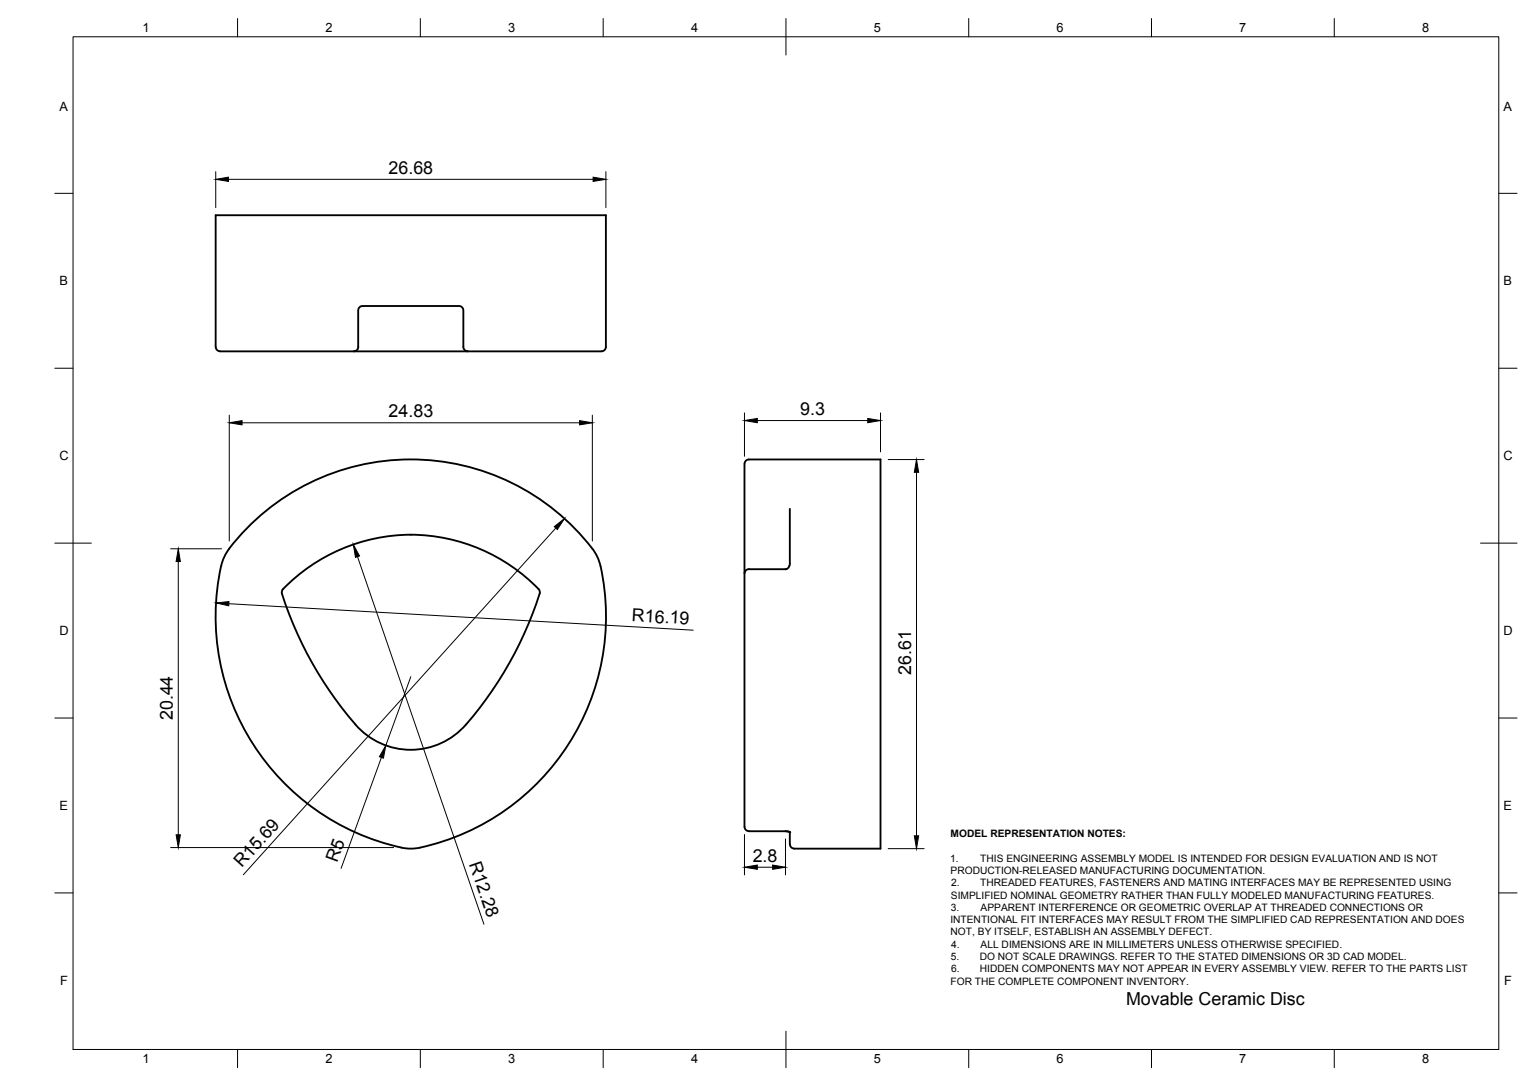
ISO-10303-21;
HEADER;
/* Generated by software containing ST-Developer
 * from STEP Tools, Inc. (www.steptools.com) 
 */

FILE_DESCRIPTION(
/* description */ ('STEP AP214'),
/* implementation_level */ '2;1');

FILE_NAME(
/* name */ 'Movable Ceramic Disc.step',
/* time_stamp */ '2026-10-06T00:19:40-07:00',
/* author */ (''),
/* organization */ (''),
/* preprocessor_version */ 'ST-DEVELOPER v20.2',
/* originating_system */ 'Autodesk Translation Framework v15.15.0.0',
/* authorisation */ '');

FILE_SCHEMA (('AUTOMOTIVE_DESIGN { 1 0 10303 214 3 1 1 }'));
ENDSEC;

DATA;
#10=MECHANICAL_DESIGN_GEOMETRIC_PRESENTATION_REPRESENTATION('',(#2071),#98302);
#411=TOROIDAL_SURFACE('',#38089,13.016744254,0.3);
#412=TOROIDAL_SURFACE('',#38103,25.2066723663,0.5);
#413=TOROIDAL_SURFACE('',#38106,11.7773059952,0.5);
#414=TOROIDAL_SURFACE('',#38114,4.5,0.5);
#415=TOROIDAL_SURFACE('',#38119,25.2066723663,0.5);
#416=TOROIDAL_SURFACE('',#38123,4.5,0.5);
#417=TOROIDAL_SURFACE('',#38131,11.7773059952,0.5);
#418=TOROIDAL_SURFACE('',#38142,13.616744254,0.3);
#419=TOROIDAL_SURFACE('',#38173,13.616744254,0.3);
#420=TOROIDAL_SURFACE('',#38197,13.7462109523,0.3);
#421=TOROIDAL_SURFACE('',#38202,2.8,0.3);
#422=TOROIDAL_SURFACE('',#38207,13.7462109523,0.3);
#423=TOROIDAL_SURFACE('',#38229,0.6,0.3);
#424=TOROIDAL_SURFACE('',#38232,13.016744254,0.3);
#425=TOROIDAL_SURFACE('',#38235,0.6,0.3);
#426=TOROIDAL_SURFACE('',#38243,0.6,0.3);
#427=TOROIDAL_SURFACE('',#38245,0.6,0.3);
#428=TOROIDAL_SURFACE('',#38253,0.6,0.3);
#429=TOROIDAL_SURFACE('',#38256,13.1462109523,0.3);
#430=TOROIDAL_SURFACE('',#38259,2.2,0.3);
#431=TOROIDAL_SURFACE('',#38262,13.1462109523,0.3);
#432=TOROIDAL_SURFACE('',#38265,0.6,0.3);
#433=TOROIDAL_SURFACE('',#38283,15.8875296363,0.3);
#434=TOROIDAL_SURFACE('',#38290,15.8875296363,0.3);
#435=TOROIDAL_SURFACE('',#38294,2.7,0.3);
#436=TOROIDAL_SURFACE('',#38307,15.8875296363,0.3);
#437=TOROIDAL_SURFACE('',#38312,15.8875296363,0.3);
#438=TOROIDAL_SURFACE('',#38317,2.7,0.3);
#439=TOROIDAL_SURFACE('',#38322,2.7,0.3);
#440=TOROIDAL_SURFACE('',#38336,15.3875296363,0.3);
#441=TOROIDAL_SURFACE('',#38338,15.3875296363,0.3);
#442=TOROIDAL_SURFACE('',#38342,15.3875296363,0.3);
#706=ELLIPSE('',#38289,0.298848923957396,0.296905362261884);
#707=ELLIPSE('',#38314,0.2988489185537,0.296905422816142);
#708=ELLIPSE('',#38324,0.298848919017662,0.29690542389071);
#709=ELLIPSE('',#38343,0.298849404757611,0.296905780207238);
#847=SPHERICAL_SURFACE('',#38146,0.3);
#848=SPHERICAL_SURFACE('',#38154,0.3);
#849=SPHERICAL_SURFACE('',#38166,0.3);
#850=SPHERICAL_SURFACE('',#38177,0.3);
#851=SPHERICAL_SURFACE('',#38195,0.3);
#852=SPHERICAL_SURFACE('',#38214,0.3);
#853=SPHERICAL_SURFACE('',#38274,0.3);
#854=SPHERICAL_SURFACE('',#38278,0.3);
#855=SPHERICAL_SURFACE('',#38298,0.3);
#856=SPHERICAL_SURFACE('',#38303,0.3);
#857=SPHERICAL_SURFACE('',#38327,0.3);
#858=SPHERICAL_SURFACE('',#38331,0.3);
#1242=B_SPLINE_SURFACE_WITH_KNOTS('',4,5,((#95885,#95886,#95887,#95888,
#95889,#95890),(#95891,#95892,#95893,#95894,#95895,#95896),(#95897,#95898,
#95899,#95900,#95901,#95902),(#95903,#95904,#95905,#95906,#95907,#95908),
(#95909,#95910,#95911,#95912,#95913,#95914)),.UNSPECIFIED.,.F.,.F.,.F.,
(5,5),(6,6),(0.,1.12670233583),(0.,0.3),.UNSPECIFIED.);
#1243=B_SPLINE_SURFACE_WITH_KNOTS('',4,5,((#96049,#96050,#96051,#96052,
#96053,#96054),(#96055,#96056,#96057,#96058,#96059,#96060),(#96061,#96062,
#96063,#96064,#96065,#96066),(#96067,#96068,#96069,#96070,#96071,#96072),
(#96073,#96074,#96075,#96076,#96077,#96078)),.UNSPECIFIED.,.F.,.F.,.F.,
(5,5),(6,6),(0.,1.12670210859),(0.,0.3),.UNSPECIFIED.);
#1244=B_SPLINE_SURFACE_WITH_KNOTS('',5,5,((#96516,#96517,#96518,#96519,
#96520,#96521,#96522,#96523,#96524),(#96525,#96526,#96527,#96528,#96529,
#96530,#96531,#96532,#96533),(#96534,#96535,#96536,#96537,#96538,#96539,
#96540,#96541,#96542),(#96543,#96544,#96545,#96546,#96547,#96548,#96549,
#96550,#96551),(#96552,#96553,#96554,#96555,#96556,#96557,#96558,#96559,
#96560),(#96561,#96562,#96563,#96564,#96565,#96566,#96567,#96568,#96569),
(#96570,#96571,#96572,#96573,#96574,#96575,#96576,#96577,#96578),(#96579,
#96580,#96581,#96582,#96583,#96584,#96585,#96586,#96587),(#96588,#96589,
#96590,#96591,#96592,#96593,#96594,#96595,#96596)),.UNSPECIFIED.,.F.,.F.,
 .F.,(6,3,6),(6,3,6),(1.82800160081,2.29147741959,2.71936718506),(0.,0.15,
0.3),.UNSPECIFIED.);
#1245=B_SPLINE_SURFACE_WITH_KNOTS('',5,5,((#96621,#96622,#96623,#96624,
#96625,#96626),(#96627,#96628,#96629,#96630,#96631,#96632),(#96633,#96634,
#96635,#96636,#96637,#96638),(#96639,#96640,#96641,#96642,#96643,#96644),
(#96645,#96646,#96647,#96648,#96649,#96650),(#96651,#96652,#96653,#96654,
#96655,#96656),(#96657,#96658,#96659,#96660,#96661,#96662),(#96663,#96664,
#96665,#96666,#96667,#96668),(#96669,#96670,#96671,#96672,#96673,#96674)),
 .UNSPECIFIED.,.F.,.F.,.F.,(6,3,6),(6,6),(1.72679799842804,2.34453942473,
2.86671715236056),(0.,0.300030052101964),.UNSPECIFIED.);
#1246=B_SPLINE_SURFACE_WITH_KNOTS('',5,5,((#96715,#96716,#96717,#96718,
#96719,#96720,#96721,#96722,#96723),(#96724,#96725,#96726,#96727,#96728,
#96729,#96730,#96731,#96732),(#96733,#96734,#96735,#96736,#96737,#96738,
#96739,#96740,#96741),(#96742,#96743,#96744,#96745,#96746,#96747,#96748,
#96749,#96750),(#96751,#96752,#96753,#96754,#96755,#96756,#96757,#96758,
#96759),(#96760,#96761,#96762,#96763,#96764,#96765,#96766,#96767,#96768),
(#96769,#96770,#96771,#96772,#96773,#96774,#96775,#96776,#96777),(#96778,
#96779,#96780,#96781,#96782,#96783,#96784,#96785,#96786),(#96787,#96788,
#96789,#96790,#96791,#96792,#96793,#96794,#96795)),.UNSPECIFIED.,.F.,.F.,
 .F.,(6,3,6),(6,3,6),(2.03426195559,2.39548583384,2.92554757),(0.,0.15,
0.3),.UNSPECIFIED.);
#1247=B_SPLINE_SURFACE_WITH_KNOTS('',5,5,((#96840,#96841,#96842,#96843,
#96844,#96845),(#96846,#96847,#96848,#96849,#96850,#96851),(#96852,#96853,
#96854,#96855,#96856,#96857),(#96858,#96859,#96860,#96861,#96862,#96863),
(#96864,#96865,#96866,#96867,#96868,#96869),(#96870,#96871,#96872,#96873,
#96874,#96875),(#96876,#96877,#96878,#96879,#96880,#96881),(#96882,#96883,
#96884,#96885,#96886,#96887),(#96888,#96889,#96890,#96891,#96892,#96893)),
 .UNSPECIFIED.,.F.,.F.,.F.,(6,3,6),(6,6),(1.66562909398,2.17637755312,2.80548129619),
(0.,0.3),.UNSPECIFIED.);
#1248=B_SPLINE_SURFACE_WITH_KNOTS('',5,5,((#96951,#96952,#96953,#96954,
#96955,#96956),(#96957,#96958,#96959,#96960,#96961,#96962),(#96963,#96964,
#96965,#96966,#96967,#96968),(#96969,#96970,#96971,#96972,#96973,#96974),
(#96975,#96976,#96977,#96978,#96979,#96980),(#96981,#96982,#96983,#96984,
#96985,#96986)),.UNSPECIFIED.,.F.,.F.,.F.,(6,6),(6,6),(1.15863824043,1.47670435084),
(0.,0.3),.UNSPECIFIED.);
#1249=B_SPLINE_SURFACE_WITH_KNOTS('',5,5,((#97008,#97009,#97010,#97011,
#97012,#97013),(#97014,#97015,#97016,#97017,#97018,#97019),(#97020,#97021,
#97022,#97023,#97024,#97025),(#97026,#97027,#97028,#97029,#97030,#97031),
(#97032,#97033,#97034,#97035,#97036,#97037),(#97038,#97039,#97040,#97041,
#97042,#97043)),.UNSPECIFIED.,.F.,.F.,.F.,(6,6),(6,6),(1.69754904882,2.01561058189),
(0.,0.3),.UNSPECIFIED.);
#1250=B_SPLINE_SURFACE_WITH_KNOTS('',5,5,((#97079,#97080,#97081,#97082,
#97083,#97084),(#97085,#97086,#97087,#97088,#97089,#97090),(#97091,#97092,
#97093,#97094,#97095,#97096),(#97097,#97098,#97099,#97100,#97101,#97102),
(#97103,#97104,#97105,#97106,#97107,#97108),(#97109,#97110,#97111,#97112,
#97113,#97114),(#97115,#97116,#97117,#97118,#97119,#97120),(#97121,#97122,
#97123,#97124,#97125,#97126),(#97127,#97128,#97129,#97130,#97131,#97132)),
 .UNSPECIFIED.,.F.,.F.,.F.,(6,3,6),(6,6),(1.64809551428,2.25520583962,2.74124708106),
(0.,0.3),.UNSPECIFIED.);
#1251=B_SPLINE_SURFACE_WITH_KNOTS('',5,5,((#97186,#97187,#97188,#97189,
#97190,#97191),(#97192,#97193,#97194,#97195,#97196,#97197),(#97198,#97199,
#97200,#97201,#97202,#97203),(#97204,#97205,#97206,#97207,#97208,#97209),
(#97210,#97211,#97212,#97213,#97214,#97215),(#97216,#97217,#97218,#97219,
#97220,#97221),(#97222,#97223,#97224,#97225,#97226,#97227),(#97228,#97229,
#97230,#97231,#97232,#97233),(#97234,#97235,#97236,#97237,#97238,#97239)),
 .UNSPECIFIED.,.F.,.F.,.F.,(6,3,6),(6,6),(1.62043318117,2.09769319653,2.71358394784),
(0.,0.3),.UNSPECIFIED.);
#1315=FACE_BOUND('',#7442,.T.);
#2003=B_SPLINE_CURVE_WITH_KNOTS('',3,(#95827,#95828,#95829,#95830,#95831,
#95832,#95833,#95834,#95835,#95836,#95837,#95838,#95839,#95840,#95841,#95842,
#95843,#95844,#95845,#95846,#95847,#95848,#95849,#95850,#95851,#95852,#95853,
#95854,#95855,#95856,#95857,#95858,#95859,#95860,#95861,#95862,#95863,#95864,
#95865,#95866,#95867,#95868,#95869,#95870,#95871,#95872,#95873,#95874,#95875,
#95876,#95877,#95878,#95879,#95880,#95881),.UNSPECIFIED.,.F.,.F.,(4,3,3,
3,3,3,3,3,3,3,3,3,3,3,3,3,3,3,4),(0.,0.12433707374752,0.236463112232104,
0.337929106180553,0.432268616281982,0.468749999999944,0.484564663314929,
0.49999999999994,0.579748767028655,0.624999999999925,0.702664260176126,
0.734374999999922,0.743377244119339,0.749999999999923,0.808401595020124,
0.863301770524771,0.915898796756716,0.96483781443388,1.),.UNSPECIFIED.);
#2004=B_SPLINE_CURVE_WITH_KNOTS('',3,(#95915,#95916,#95917,#95918,#95919,
#95920,#95921,#95922,#95923,#95924,#95925,#95926,#95927,#95928,#95929,#95930,
#95931,#95932,#95933,#95934,#95935,#95936,#95937,#95938,#95939,#95940,#95941,
#95942,#95943,#95944,#95945),.UNSPECIFIED.,.F.,.F.,(4,3,3,3,3,3,3,3,3,3,
4),(0.,0.100659233418489,0.201318874239452,0.301978728327487,0.402638920630661,
0.5,0.599561871286431,0.699671403464823,0.800121822811729,0.903065513154291,
1.),.UNSPECIFIED.);
#2005=B_SPLINE_CURVE_WITH_KNOTS('',4,(#95968,#95969,#95970,#95971,#95972),
 .UNSPECIFIED.,.F.,.F.,(5,5),(0.,1.),.UNSPECIFIED.);
#2006=B_SPLINE_CURVE_WITH_KNOTS('',3,(#95993,#95994,#95995,#95996,#95997,
#95998,#95999,#96000,#96001,#96002,#96003,#96004,#96005,#96006,#96007,#96008,
#96009,#96010,#96011,#96012,#96013,#96014,#96015,#96016,#96017,#96018,#96019,
#96020,#96021,#96022,#96023,#96024,#96025,#96026,#96027,#96028,#96029,#96030,
#96031,#96032,#96033,#96034,#96035,#96036,#96037,#96038,#96039,#96040,#96041,
#96042,#96043,#96044,#96045,#96046,#96047),.UNSPECIFIED.,.F.,.F.,(4,3,3,
3,3,3,3,3,3,3,3,3,3,3,3,3,3,3,4),(0.,0.126260093452782,0.241158460346812,
0.339992840904553,0.437500000000044,0.468750000000048,0.484662798051363,
0.500000000000052,0.580119369937759,0.625000000000081,0.70316841264024,
0.734375000000096,0.743449522410721,0.750000000000096,0.809065654268961,
0.864511341100943,0.917619180392791,0.9671021347712,1.),.UNSPECIFIED.);
#2007=B_SPLINE_CURVE_WITH_KNOTS('',5,(#96095,#96096,#96097,#96098,#96099,
#96100,#96101,#96102,#96103,#96104,#96105,#96106,#96107,#96108,#96109,#96110,
#96111,#96112),.UNSPECIFIED.,.F.,.F.,(6,3,3,3,3,6),(2.03426195559,2.39548583384,
2.56639489646,2.72897717597,2.88469745612,2.92554757),.UNSPECIFIED.);
#2008=B_SPLINE_CURVE_WITH_KNOTS('',3,(#96113,#96114,#96115,#96116,#96117,
#96118,#96119,#96120,#96121,#96122),.UNSPECIFIED.,.F.,.F.,(4,3,3,4),(1.69754904882,
1.84161408159244,1.88420275149,2.01561058189),.UNSPECIFIED.);
#2009=B_SPLINE_CURVE_WITH_KNOTS('',3,(#96150,#96151,#96152,#96153,#96154,
#96155,#96156,#96157,#96158,#96159,#96160,#96161,#96162,#96163,#96164,#96165,
#96166,#96167,#96168,#96169,#96170,#96171,#96172,#96173,#96174,#96175,#96176,
#96177,#96178,#96179,#96180,#96181,#96182,#96183,#96184,#96185,#96186),
 .UNSPECIFIED.,.F.,.F.,(4,3,3,3,3,3,3,3,3,3,3,3,4),(1.64809551428,1.7475192804611,
1.85317562308383,1.96283960328877,2.07841864168069,2.10047189796,2.21451207594883,
2.25520583962,2.38637299327516,2.52642486466674,2.57088104253,2.72494913183819,
2.74124708106),.UNSPECIFIED.);
#2010=B_SPLINE_CURVE_WITH_KNOTS('',5,(#96213,#96214,#96215,#96216,#96217,
#96218,#96219,#96220,#96221),.UNSPECIFIED.,.F.,.F.,(6,3,6),(0.,0.436591209475934,
1.),.UNSPECIFIED.);
#2011=B_SPLINE_CURVE_WITH_KNOTS('',3,(#96246,#96247,#96248,#96249,#96250,
#96251,#96252,#96253,#96254,#96255),.UNSPECIFIED.,.F.,.F.,(4,3,3,4),(1.15863824043,
1.30484728031855,1.3519323715,1.47670435084),.UNSPECIFIED.);
#2012=B_SPLINE_CURVE_WITH_KNOTS('',5,(#96257,#96258,#96259,#96260,#96261,
#96262,#96263,#96264,#96265,#96266,#96267,#96268,#96269,#96270,#96271),
 .UNSPECIFIED.,.F.,.F.,(6,3,3,3,6),(1.82800160081,2.13151904383,2.29147741959,
2.45912256669,2.71936718506),.UNSPECIFIED.);
#2013=B_SPLINE_CURVE_WITH_KNOTS('',3,(#96296,#96297,#96298,#96299,#96300,
#96301,#96302,#96303,#96304,#96305,#96306,#96307,#96308,#96309,#96310,#96311,
#96312,#96313,#96314,#96315,#96316,#96317,#96318,#96319,#96320,#96321,#96322,
#96323,#96324,#96325,#96326,#96327,#96328,#96329),.UNSPECIFIED.,.F.,.F.,
(4,3,3,3,3,3,3,3,3,3,3,4),(1.72682805053,1.82706316337451,1.92770774168372,
2.02823087921,2.14486360402001,2.18407667554,2.31552494470154,2.34453942473,
2.49244062175995,2.50972074403,2.678720463,2.86668722779),.UNSPECIFIED.);
#2014=B_SPLINE_CURVE_WITH_KNOTS('',5,(#96381,#96382,#96383,#96384,#96385,
#96386,#96387,#96388,#96389,#96390,#96391,#96392,#96393,#96394,#96395,#96396,
#96397,#96398,#96399,#96400,#96401),.UNSPECIFIED.,.F.,.F.,(6,3,3,3,3,3,
6),(1.66562909398,1.83574953953,2.17637755312,2.34189323073,2.50257634582,
2.65848585647,2.80548129619),.UNSPECIFIED.);
#2015=B_SPLINE_CURVE_WITH_KNOTS('',5,(#96601,#96602,#96603,#96604,#96605,
#96606,#96607,#96608,#96609),.UNSPECIFIED.,.F.,.F.,(6,3,6),(1.82800160081,
2.29147741959,2.71936718506),.UNSPECIFIED.);
#2016=B_SPLINE_CURVE_WITH_KNOTS('',5,(#96615,#96616,#96617,#96618,#96619,
#96620),.UNSPECIFIED.,.F.,.F.,(6,6),(0.,1.),.UNSPECIFIED.);
#2017=B_SPLINE_CURVE_WITH_KNOTS('',5,(#96676,#96677,#96678,#96679,#96680,
#96681,#96682,#96683,#96684),.UNSPECIFIED.,.F.,.F.,(6,3,6),(0.,0.541919025194724,
1.),.UNSPECIFIED.);
#2018=B_SPLINE_CURVE_WITH_KNOTS('',3,(#96800,#96801,#96802,#96803,#96804,
#96805,#96806,#96807,#96808,#96809,#96810,#96811,#96812,#96813,#96814,#96815,
#96816,#96817,#96818,#96819,#96820,#96821,#96822,#96823,#96824,#96825,#96826,
#96827,#96828,#96829,#96830,#96831,#96832,#96833),.UNSPECIFIED.,.F.,.F.,
(4,3,3,3,3,3,3,3,3,3,3,4),(2.03426195559,2.1510096123002,2.25715585151842,
2.35241102166568,2.39548582166195,2.47480008629705,2.55703499531236,2.6389374730589,
2.71532446519286,2.78841164259849,2.85704870664929,2.92554757),
 .UNSPECIFIED.);
#2019=B_SPLINE_CURVE_WITH_KNOTS('',5,(#96895,#96896,#96897,#96898,#96899,
#96900,#96901,#96902,#96903),.UNSPECIFIED.,.F.,.F.,(6,3,6),(0.,0.44808305686451,
1.),.UNSPECIFIED.);
#2020=B_SPLINE_CURVE_WITH_KNOTS('',3,(#96904,#96905,#96906,#96907,#96908,
#96909,#96910,#96911,#96912,#96913,#96914,#96915,#96916,#96917,#96918,#96919,
#96920,#96921,#96922,#96923,#96924,#96925,#96926,#96927,#96928,#96929,#96930,
#96931,#96932,#96933,#96934,#96935,#96936,#96937,#96938,#96939,#96940),
 .UNSPECIFIED.,.F.,.F.,(4,3,3,3,3,3,3,3,3,3,3,3,4),(0.,0.0846906362845857,
0.170916588348621,0.259457677757533,0.349118725584472,0.440002922090847,
0.5,0.590971966453158,0.681170088206319,0.76944906347906,0.856421296291944,
0.941305445099306,1.),.UNSPECIFIED.);
#2021=B_SPLINE_CURVE_WITH_KNOTS('',3,(#96987,#96988,#96989,#96990,#96991,
#96992,#96993,#96994,#96995,#96996,#96997,#96998,#96999),.UNSPECIFIED.,
 .F.,.F.,(4,3,3,3,4),(0.,0.307479208897056,0.622231708274825,0.935862006693834,
1.),.UNSPECIFIED.);
#2022=B_SPLINE_CURVE_WITH_KNOTS('',3,(#97044,#97045,#97046,#97047,#97048,
#97049,#97050,#97051,#97052,#97053,#97054,#97055,#97056),.UNSPECIFIED.,
 .F.,.F.,(4,3,3,3,4),(0.,0.314421563164034,0.629924180845976,0.934742918075105,
1.),.UNSPECIFIED.);
#2023=B_SPLINE_CURVE_WITH_KNOTS('',5,(#97134,#97135,#97136,#97137,#97138,
#97139),.UNSPECIFIED.,.F.,.F.,(6,6),(0.,1.),.UNSPECIFIED.);
#2024=B_SPLINE_CURVE_WITH_KNOTS('',3,(#97140,#97141,#97142,#97143,#97144,
#97145,#97146,#97147,#97148,#97149,#97150,#97151,#97152,#97153,#97154,#97155,
#97156,#97157,#97158,#97159,#97160,#97161,#97162,#97163,#97164,#97165,#97166,
#97167,#97168,#97169,#97170,#97171,#97172,#97173,#97174,#97175,#97176,#97177,
#97178,#97179),.UNSPECIFIED.,.F.,.F.,(4,3,3,3,3,3,3,3,3,3,3,3,3,4),(0.,
0.0817493380761543,0.167757777444047,0.260434121556351,0.356347053996799,
0.453676990608725,0.500000000000004,0.555446107885843,0.657734231357899,
0.750000000000002,0.824982076180982,0.899805956993093,0.97269336693032,
1.),.UNSPECIFIED.);
#2025=B_SPLINE_CURVE_WITH_KNOTS('',3,(#97241,#97242,#97243,#97244,#97245,
#97246,#97247,#97248,#97249,#97250,#97251,#97252,#97253,#97254,#97255,#97256,
#97257,#97258,#97259,#97260,#97261,#97262,#97263,#97264,#97265,#97266,#97267,
#97268,#97269,#97270,#97271,#97272,#97273,#97274),.UNSPECIFIED.,.F.,.F.,
(4,3,3,3,3,3,3,3,3,3,3,4),(0.,0.0958054567289393,0.193447450982335,0.294266519609543,
0.395565390771468,0.499287123804762,0.59780946855357,0.698357101415177,
0.797410250015008,0.898705125007504,0.994263256631534,1.),.UNSPECIFIED.);
#2026=B_SPLINE_CURVE_WITH_KNOTS('',3,(#97275,#97276,#97277,#97278,#97279,
#97280,#97281,#97282,#97283,#97284,#97285,#97286,#97287,#97288,#97289,#97290,
#97291,#97292,#97293,#97294,#97295,#97296,#97297,#97298,#97299,#97300,#97301,
#97302,#97303,#97304,#97305,#97306,#97307,#97308,#97309,#97310,#97311,#97312,
#97313,#97314,#97315,#97316,#97317,#97318,#97319,#97320,#97321,#97322,#97323,
#97324,#97325,#97326),.UNSPECIFIED.,.F.,.F.,(4,3,3,3,3,3,3,3,3,3,3,3,3,
3,3,3,3,4),(0.,0.0625,0.125471806190554,0.187993683396628,0.25,0.312017100075837,
0.374475387343952,0.436933674612067,0.5,0.5625,0.623237451244149,0.683323686394024,
0.741866361912494,0.75,0.819559695460738,0.889734230242426,0.959282737790169,
1.),.UNSPECIFIED.);
#2051=SHAPE_REPRESENTATION_RELATIONSHIP('SRR','None',#98348,#2061);
#2061=ADVANCED_BREP_SHAPE_REPRESENTATION('',(#2080),#98300);
#2071=STYLED_ITEM('',(#98399),#2080);
#2080=MANIFOLD_SOLID_BREP('Body1',#34177);
#2440=PLANE('',#38109);
#2441=PLANE('',#38135);
#2442=PLANE('',#38141);
#2443=PLANE('',#38158);
#2444=PLANE('',#38159);
#2445=PLANE('',#38165);
#2446=PLANE('',#38181);
#2447=PLANE('',#38182);
#2448=PLANE('',#38185);
#2449=PLANE('',#38218);
#2450=PLANE('',#38219);
#2451=PLANE('',#38270);
#3191=CYLINDRICAL_SURFACE('',#38094,25.7066723663);
#3192=CYLINDRICAL_SURFACE('',#38097,0.3);
#3193=CYLINDRICAL_SURFACE('',#38100,12.2773059952);
#3194=CYLINDRICAL_SURFACE('',#38117,5.);
#3195=CYLINDRICAL_SURFACE('',#38121,25.7066723663);
#3196=CYLINDRICAL_SURFACE('',#38126,5.);
#3197=CYLINDRICAL_SURFACE('',#38128,0.3);
#3198=CYLINDRICAL_SURFACE('',#38133,12.2773059952);
#3199=CYLINDRICAL_SURFACE('',#38139,0.300000000000002);
#3200=CYLINDRICAL_SURFACE('',#38148,0.300000000000001);
#3201=CYLINDRICAL_SURFACE('',#38150,13.316744254);
#3202=CYLINDRICAL_SURFACE('',#38152,0.3);
#3203=CYLINDRICAL_SURFACE('',#38156,0.3);
#3204=CYLINDRICAL_SURFACE('',#38163,0.300000000000002);
#3205=CYLINDRICAL_SURFACE('',#38169,0.3);
#3206=CYLINDRICAL_SURFACE('',#38171,13.316744254);
#3207=CYLINDRICAL_SURFACE('',#38175,0.3);
#3208=CYLINDRICAL_SURFACE('',#38179,0.300000000000001);
#3209=CYLINDRICAL_SURFACE('',#38183,0.300000000000002);
#3210=CYLINDRICAL_SURFACE('',#38192,0.3);
#3211=CYLINDRICAL_SURFACE('',#38200,13.4462109523);
#3212=CYLINDRICAL_SURFACE('',#38205,2.5);
#3213=CYLINDRICAL_SURFACE('',#38210,13.4462109523);
#3214=CYLINDRICAL_SURFACE('',#38212,0.3);
#3215=CYLINDRICAL_SURFACE('',#38216,0.3);
#3216=CYLINDRICAL_SURFACE('',#38226,0.300000000000002);
#3217=CYLINDRICAL_SURFACE('',#38238,0.3);
#3218=CYLINDRICAL_SURFACE('',#38240,0.300000000000002);
#3219=CYLINDRICAL_SURFACE('',#38248,0.3);
#3220=CYLINDRICAL_SURFACE('',#38250,0.300000000000002);
#3221=CYLINDRICAL_SURFACE('',#38268,0.3);
#3222=CYLINDRICAL_SURFACE('',#38287,0.3);
#3223=CYLINDRICAL_SURFACE('',#38288,0.3);
#3224=CYLINDRICAL_SURFACE('',#38293,16.1875296363);
#3225=CYLINDRICAL_SURFACE('',#38297,3.);
#3226=CYLINDRICAL_SURFACE('',#38311,0.3);
#3227=CYLINDRICAL_SURFACE('',#38315,0.299999999999999);
#3228=CYLINDRICAL_SURFACE('',#38316,16.1875296363);
#3229=CYLINDRICAL_SURFACE('',#38321,3.);
#3230=CYLINDRICAL_SURFACE('',#38326,3.);
#3231=CYLINDRICAL_SURFACE('',#38341,0.3);
#3232=CYLINDRICAL_SURFACE('',#38345,0.3);
#3233=CYLINDRICAL_SURFACE('',#38346,15.6875296363);
#5185=FACE_OUTER_BOUND('',#7386,.T.);
#5186=FACE_OUTER_BOUND('',#7387,.T.);
#5187=FACE_OUTER_BOUND('',#7388,.T.);
#5188=FACE_OUTER_BOUND('',#7389,.T.);
#5189=FACE_OUTER_BOUND('',#7390,.T.);
#5190=FACE_OUTER_BOUND('',#7391,.T.);
#5191=FACE_OUTER_BOUND('',#7392,.T.);
#5192=FACE_OUTER_BOUND('',#7393,.T.);
#5193=FACE_OUTER_BOUND('',#7394,.T.);
#5194=FACE_OUTER_BOUND('',#7395,.T.);
#5195=FACE_OUTER_BOUND('',#7396,.T.);
#5196=FACE_OUTER_BOUND('',#7397,.T.);
#5197=FACE_OUTER_BOUND('',#7398,.T.);
#5198=FACE_OUTER_BOUND('',#7399,.T.);
#5199=FACE_OUTER_BOUND('',#7400,.T.);
#5200=FACE_OUTER_BOUND('',#7401,.T.);
#5201=FACE_OUTER_BOUND('',#7402,.T.);
#5202=FACE_OUTER_BOUND('',#7403,.T.);
#5203=FACE_OUTER_BOUND('',#7404,.T.);
#5204=FACE_OUTER_BOUND('',#7405,.T.);
#5205=FACE_OUTER_BOUND('',#7406,.T.);
#5206=FACE_OUTER_BOUND('',#7407,.T.);
#5207=FACE_OUTER_BOUND('',#7408,.T.);
#5208=FACE_OUTER_BOUND('',#7409,.T.);
#5209=FACE_OUTER_BOUND('',#7410,.T.);
#5210=FACE_OUTER_BOUND('',#7411,.T.);
#5211=FACE_OUTER_BOUND('',#7412,.T.);
#5212=FACE_OUTER_BOUND('',#7413,.T.);
#5213=FACE_OUTER_BOUND('',#7414,.T.);
#5214=FACE_OUTER_BOUND('',#7415,.T.);
#5215=FACE_OUTER_BOUND('',#7416,.T.);
#5216=FACE_OUTER_BOUND('',#7417,.T.);
#5217=FACE_OUTER_BOUND('',#7418,.T.);
#5218=FACE_OUTER_BOUND('',#7419,.T.);
#5219=FACE_OUTER_BOUND('',#7420,.T.);
#5220=FACE_OUTER_BOUND('',#7421,.T.);
#5221=FACE_OUTER_BOUND('',#7422,.T.);
#5222=FACE_OUTER_BOUND('',#7423,.T.);
#5223=FACE_OUTER_BOUND('',#7424,.T.);
#5224=FACE_OUTER_BOUND('',#7425,.T.);
#5225=FACE_OUTER_BOUND('',#7426,.T.);
#5226=FACE_OUTER_BOUND('',#7427,.T.);
#5227=FACE_OUTER_BOUND('',#7428,.T.);
#5228=FACE_OUTER_BOUND('',#7429,.T.);
#5229=FACE_OUTER_BOUND('',#7430,.T.);
#5230=FACE_OUTER_BOUND('',#7431,.T.);
#5231=FACE_OUTER_BOUND('',#7432,.T.);
#5232=FACE_OUTER_BOUND('',#7433,.T.);
#5233=FACE_OUTER_BOUND('',#7434,.T.);
#5234=FACE_OUTER_BOUND('',#7435,.T.);
#5235=FACE_OUTER_BOUND('',#7436,.T.);
#5236=FACE_OUTER_BOUND('',#7437,.T.);
#5237=FACE_OUTER_BOUND('',#7438,.T.);
#5238=FACE_OUTER_BOUND('',#7439,.T.);
#5239=FACE_OUTER_BOUND('',#7440,.T.);
#5240=FACE_OUTER_BOUND('',#7441,.T.);
#5241=FACE_OUTER_BOUND('',#7443,.T.);
#5242=FACE_OUTER_BOUND('',#7444,.T.);
#5243=FACE_OUTER_BOUND('',#7445,.T.);
#5244=FACE_OUTER_BOUND('',#7446,.T.);
#5245=FACE_OUTER_BOUND('',#7447,.T.);
#5246=FACE_OUTER_BOUND('',#7448,.T.);
#5247=FACE_OUTER_BOUND('',#7449,.T.);
#5248=FACE_OUTER_BOUND('',#7450,.T.);
#5249=FACE_OUTER_BOUND('',#7451,.T.);
#5250=FACE_OUTER_BOUND('',#7452,.T.);
#5251=FACE_OUTER_BOUND('',#7453,.T.);
#5252=FACE_OUTER_BOUND('',#7454,.T.);
#5253=FACE_OUTER_BOUND('',#7455,.T.);
#5254=FACE_OUTER_BOUND('',#7456,.T.);
#5255=FACE_OUTER_BOUND('',#7457,.T.);
#5256=FACE_OUTER_BOUND('',#7458,.T.);
#5257=FACE_OUTER_BOUND('',#7459,.T.);
#5258=FACE_OUTER_BOUND('',#7460,.T.);
#5259=FACE_OUTER_BOUND('',#7461,.T.);
#5260=FACE_OUTER_BOUND('',#7462,.T.);
#5261=FACE_OUTER_BOUND('',#7463,.T.);
#5262=FACE_OUTER_BOUND('',#7464,.T.);
#5263=FACE_OUTER_BOUND('',#7465,.T.);
#5264=FACE_OUTER_BOUND('',#7466,.T.);
#5265=FACE_OUTER_BOUND('',#7467,.T.);
#5266=FACE_OUTER_BOUND('',#7468,.T.);
#5267=FACE_OUTER_BOUND('',#7469,.T.);
#5268=FACE_OUTER_BOUND('',#7470,.T.);
#5269=FACE_OUTER_BOUND('',#7471,.T.);
#5270=FACE_OUTER_BOUND('',#7472,.T.);
#5271=FACE_OUTER_BOUND('',#7473,.T.);
#5272=FACE_OUTER_BOUND('',#7474,.T.);
#5273=FACE_OUTER_BOUND('',#7475,.T.);
#5274=FACE_OUTER_BOUND('',#7476,.T.);
#5275=FACE_OUTER_BOUND('',#7477,.T.);
#5276=FACE_OUTER_BOUND('',#7478,.T.);
#5277=FACE_OUTER_BOUND('',#7479,.T.);
#5278=FACE_OUTER_BOUND('',#7480,.T.);
#5279=FACE_OUTER_BOUND('',#7481,.T.);
#5280=FACE_OUTER_BOUND('',#7482,.T.);
#5281=FACE_OUTER_BOUND('',#7483,.T.);
#5282=FACE_OUTER_BOUND('',#7484,.T.);
#5283=FACE_OUTER_BOUND('',#7485,.T.);
#5284=FACE_OUTER_BOUND('',#7486,.T.);
#5285=FACE_OUTER_BOUND('',#7487,.T.);
#5286=FACE_OUTER_BOUND('',#7488,.T.);
#5287=FACE_OUTER_BOUND('',#7489,.T.);
#5288=FACE_OUTER_BOUND('',#7490,.T.);
#5289=FACE_OUTER_BOUND('',#7491,.T.);
#5290=FACE_OUTER_BOUND('',#7492,.T.);
#5291=FACE_OUTER_BOUND('',#7493,.T.);
#5292=FACE_OUTER_BOUND('',#7494,.T.);
#5293=FACE_OUTER_BOUND('',#7495,.T.);
#7386=EDGE_LOOP('',(#30841,#30842,#30843,#30844));
#7387=EDGE_LOOP('',(#30845,#30846,#30847,#30848));
#7388=EDGE_LOOP('',(#30849,#30850,#30851,#30852));
#7389=EDGE_LOOP('',(#30853,#30854,#30855,#30856));
#7390=EDGE_LOOP('',(#30857,#30858,#30859,#30860));
#7391=EDGE_LOOP('',(#30861,#30862,#30863));
#7392=EDGE_LOOP('',(#30864,#30865,#30866,#30867));
#7393=EDGE_LOOP('',(#30868,#30869,#30870,#30871,#30872,#30873));
#7394=EDGE_LOOP('',(#30874,#30875,#30876,#30877));
#7395=EDGE_LOOP('',(#30878,#30879,#30880,#30881));
#7396=EDGE_LOOP('',(#30882,#30883,#30884,#30885));
#7397=EDGE_LOOP('',(#30886,#30887,#30888,#30889));
#7398=EDGE_LOOP('',(#30890,#30891,#30892,#30893));
#7399=EDGE_LOOP('',(#30894,#30895,#30896,#30897));
#7400=EDGE_LOOP('',(#30898,#30899,#30900,#30901));
#7401=EDGE_LOOP('',(#30902,#30903,#30904,#30905));
#7402=EDGE_LOOP('',(#30906,#30907,#30908));
#7403=EDGE_LOOP('',(#30909,#30910,#30911,#30912));
#7404=EDGE_LOOP('',(#30913,#30914,#30915,#30916,#30917));
#7405=EDGE_LOOP('',(#30918,#30919,#30920,#30921,#30922));
#7406=EDGE_LOOP('',(#30923,#30924,#30925,#30926));
#7407=EDGE_LOOP('',(#30927,#30928,#30929,#30930));
#7408=EDGE_LOOP('',(#30931,#30932,#30933));
#7409=EDGE_LOOP('',(#30934,#30935,#30936,#30937));
#7410=EDGE_LOOP('',(#30938,#30939,#30940,#30941));
#7411=EDGE_LOOP('',(#30942,#30943,#30944,#30945));
#7412=EDGE_LOOP('',(#30946,#30947,#30948));
#7413=EDGE_LOOP('',(#30949,#30950,#30951,#30952));
#7414=EDGE_LOOP('',(#30953,#30954,#30955,#30956));
#7415=EDGE_LOOP('',(#30957,#30958,#30959,#30960,#30961));
#7416=EDGE_LOOP('',(#30962,#30963,#30964,#30965));
#7417=EDGE_LOOP('',(#30966,#30967,#30968,#30969));
#7418=EDGE_LOOP('',(#30970,#30971,#30972));
#7419=EDGE_LOOP('',(#30973,#30974,#30975,#30976));
#7420=EDGE_LOOP('',(#30977,#30978,#30979,#30980));
#7421=EDGE_LOOP('',(#30981,#30982,#30983,#30984));
#7422=EDGE_LOOP('',(#30985,#30986,#30987,#30988,#30989));
#7423=EDGE_LOOP('',(#30990,#30991,#30992));
#7424=EDGE_LOOP('',(#30993,#30994,#30995,#30996));
#7425=EDGE_LOOP('',(#30997,#30998,#30999,#31000));
#7426=EDGE_LOOP('',(#31001,#31002,#31003,#31004));
#7427=EDGE_LOOP('',(#31005,#31006,#31007,#31008));
#7428=EDGE_LOOP('',(#31009,#31010,#31011,#31012,#31013,#31014,#31015,#31016));
#7429=EDGE_LOOP('',(#31017,#31018,#31019,#31020));
#7430=EDGE_LOOP('',(#31021,#31022,#31023));
#7431=EDGE_LOOP('',(#31024,#31025,#31026,#31027));
#7432=EDGE_LOOP('',(#31028,#31029,#31030,#31031));
#7433=EDGE_LOOP('',(#31032,#31033,#31034,#31035));
#7434=EDGE_LOOP('',(#31036,#31037,#31038,#31039));
#7435=EDGE_LOOP('',(#31040,#31041,#31042,#31043));
#7436=EDGE_LOOP('',(#31044,#31045,#31046,#31047));
#7437=EDGE_LOOP('',(#31048,#31049,#31050,#31051));
#7438=EDGE_LOOP('',(#31052,#31053,#31054));
#7439=EDGE_LOOP('',(#31055,#31056,#31057,#31058));
#7440=EDGE_LOOP('',(#31059,#31060,#31061,#31062));
#7441=EDGE_LOOP('',(#31063,#31064,#31065,#31066,#31067,#31068));
#7442=EDGE_LOOP('',(#31069,#31070,#31071,#31072,#31073,#31074,#31075,#31076));
#7443=EDGE_LOOP('',(#31077,#31078,#31079,#31080));
#7444=EDGE_LOOP('',(#31081,#31082,#31083,#31084));
#7445=EDGE_LOOP('',(#31085,#31086,#31087,#31088));
#7446=EDGE_LOOP('',(#31089,#31090,#31091,#31092));
#7447=EDGE_LOOP('',(#31093,#31094,#31095,#31096));
#7448=EDGE_LOOP('',(#31097,#31098,#31099,#31100));
#7449=EDGE_LOOP('',(#31101,#31102,#31103,#31104));
#7450=EDGE_LOOP('',(#31105,#31106,#31107,#31108));
#7451=EDGE_LOOP('',(#31109,#31110,#31111,#31112));
#7452=EDGE_LOOP('',(#31113,#31114,#31115,#31116));
#7453=EDGE_LOOP('',(#31117,#31118,#31119,#31120));
#7454=EDGE_LOOP('',(#31121,#31122,#31123,#31124));
#7455=EDGE_LOOP('',(#31125,#31126,#31127,#31128));
#7456=EDGE_LOOP('',(#31129,#31130,#31131,#31132));
#7457=EDGE_LOOP('',(#31133,#31134,#31135,#31136));
#7458=EDGE_LOOP('',(#31137,#31138,#31139,#31140));
#7459=EDGE_LOOP('',(#31141,#31142,#31143,#31144,#31145,#31146,#31147,#31148,
#31149,#31150,#31151,#31152,#31153,#31154,#31155,#31156,#31157,#31158,#31159,
#31160));
#7460=EDGE_LOOP('',(#31161,#31162,#31163,#31164,#31165));
#7461=EDGE_LOOP('',(#31166,#31167,#31168,#31169,#31170,#31171));
#7462=EDGE_LOOP('',(#31172,#31173,#31174,#31175));
#7463=EDGE_LOOP('',(#31176,#31177,#31178,#31179));
#7464=EDGE_LOOP('',(#31180,#31181,#31182,#31183));
#7465=EDGE_LOOP('',(#31184,#31185,#31186,#31187,#31188));
#7466=EDGE_LOOP('',(#31189,#31190,#31191,#31192));
#7467=EDGE_LOOP('',(#31193,#31194,#31195,#31196));
#7468=EDGE_LOOP('',(#31197,#31198,#31199,#31200,#31201,#31202,#31203,#31204,
#31205));
#7469=EDGE_LOOP('',(#31206,#31207,#31208,#31209));
#7470=EDGE_LOOP('',(#31210,#31211,#31212,#31213));
#7471=EDGE_LOOP('',(#31214,#31215,#31216,#31217,#31218,#31219));
#7472=EDGE_LOOP('',(#31220,#31221,#31222,#31223,#31224));
#7473=EDGE_LOOP('',(#31225,#31226,#31227,#31228));
#7474=EDGE_LOOP('',(#31229,#31230,#31231,#31232));
#7475=EDGE_LOOP('',(#31233,#31234,#31235,#31236,#31237));
#7476=EDGE_LOOP('',(#31238,#31239,#31240,#31241));
#7477=EDGE_LOOP('',(#31242,#31243,#31244,#31245));
#7478=EDGE_LOOP('',(#31246,#31247,#31248,#31249));
#7479=EDGE_LOOP('',(#31250,#31251,#31252,#31253,#31254,#31255,#31256,#31257,
#31258));
#7480=EDGE_LOOP('',(#31259,#31260,#31261,#31262));
#7481=EDGE_LOOP('',(#31263,#31264,#31265,#31266));
#7482=EDGE_LOOP('',(#31267,#31268,#31269,#31270,#31271));
#7483=EDGE_LOOP('',(#31272,#31273,#31274,#31275));
#7484=EDGE_LOOP('',(#31276,#31277,#31278,#31279));
#7485=EDGE_LOOP('',(#31280,#31281,#31282,#31283,#31284));
#7486=EDGE_LOOP('',(#31285,#31286,#31287,#31288,#31289));
#7487=EDGE_LOOP('',(#31290,#31291,#31292,#31293,#31294,#31295));
#7488=EDGE_LOOP('',(#31296,#31297,#31298,#31299));
#7489=EDGE_LOOP('',(#31300,#31301,#31302,#31303));
#7490=EDGE_LOOP('',(#31304,#31305,#31306,#31307));
#7491=EDGE_LOOP('',(#31308,#31309,#31310,#31311));
#7492=EDGE_LOOP('',(#31312,#31313,#31314,#31315));
#7493=EDGE_LOOP('',(#31316,#31317,#31318,#31319));
#7494=EDGE_LOOP('',(#31320,#31321,#31322,#31323,#31324));
#7495=EDGE_LOOP('',(#31325,#31326,#31327,#31328,#31329,#31330,#31331,#31332,
#31333,#31334));
#9220=LINE('',#95809,#11060);
#9221=LINE('',#95812,#11061);
#9222=LINE('',#95818,#11062);
#9223=LINE('',#95824,#11063);
#9224=LINE('',#95964,#11064);
#9225=LINE('',#95976,#11065);
#9226=LINE('',#95985,#11066);
#9227=LINE('',#95990,#11067);
#9228=LINE('',#96084,#11068);
#9229=LINE('',#96088,#11069);
#9230=LINE('',#96125,#11070);
#9231=LINE('',#96129,#11071);
#9232=LINE('',#96130,#11072);
#9233=LINE('',#96131,#11073);
#9234=LINE('',#96143,#11074);
#9235=LINE('',#96146,#11075);
#9236=LINE('',#96188,#11076);
#9237=LINE('',#96195,#11077);
#9238=LINE('',#96198,#11078);
#9239=LINE('',#96199,#11079);
#9240=LINE('',#96203,#11080);
#9241=LINE('',#96207,#11081);
#9242=LINE('',#96224,#11082);
#9243=LINE('',#96228,#11083);
#9244=LINE('',#96229,#11084);
#9245=LINE('',#96230,#11085);
#9246=LINE('',#96237,#11086);
#9247=LINE('',#96241,#11087);
#9248=LINE('',#96273,#11088);
#9249=LINE('',#96280,#11089);
#9250=LINE('',#96283,#11090);
#9251=LINE('',#96284,#11091);
#9252=LINE('',#96288,#11092);
#9253=LINE('',#96290,#11093);
#9254=LINE('',#96292,#11094);
#9255=LINE('',#96293,#11095);
#9256=LINE('',#96331,#11096);
#9257=LINE('',#96336,#11097);
#9258=LINE('',#96352,#11098);
#9259=LINE('',#96361,#11099);
#9260=LINE('',#96369,#11100);
#9261=LINE('',#96377,#11101);
#9262=LINE('',#96403,#11102);
#9263=LINE('',#96410,#11103);
#9264=LINE('',#96413,#11104);
#9265=LINE('',#96414,#11105);
#9266=LINE('',#96433,#11106);
#9267=LINE('',#96449,#11107);
#9268=LINE('',#96455,#11108);
#9269=LINE('',#96465,#11109);
#9270=LINE('',#96470,#11110);
#9271=LINE('',#96495,#11111);
#9272=LINE('',#96611,#11112);
#9273=LINE('',#96614,#11113);
#9274=LINE('',#96691,#11114);
#9275=LINE('',#96692,#11115);
#9276=LINE('',#96698,#11116);
#9277=LINE('',#96835,#11117);
#9278=LINE('',#96942,#11118);
#9279=LINE('',#96944,#11119);
#9280=LINE('',#97001,#11120);
#9281=LINE('',#97058,#11121);
#9282=LINE('',#97181,#11122);
#9283=LINE('',#97328,#11123);
#11060=VECTOR('',#47811,1000.);
#11061=VECTOR('',#47814,1000.);
#11062=VECTOR('',#47821,1000.);
#11063=VECTOR('',#47828,1000.);
#11064=VECTOR('',#47859,1000.);
#11065=VECTOR('',#47868,1000.);
#11066=VECTOR('',#47881,1000.);
#11067=VECTOR('',#47886,1000.);
#11068=VECTOR('',#47899,1000.);
#11069=VECTOR('',#47902,1000.);
#11070=VECTOR('',#47911,1000.);
#11071=VECTOR('',#47914,1000.);
#11072=VECTOR('',#47915,1000.);
#11073=VECTOR('',#47916,1000.);
#11074=VECTOR('',#47933,1000.);
#11075=VECTOR('',#47936,1000.);
#11076=VECTOR('',#47941,1000.);
#11077=VECTOR('',#47952,1000.);
#11078=VECTOR('',#47955,1000.);
#11079=VECTOR('',#47956,1000.);
#11080=VECTOR('',#47959,1000.);
#11081=VECTOR('',#47962,1000.);
#11082=VECTOR('',#47971,1000.);
#11083=VECTOR('',#47974,1000.);
#11084=VECTOR('',#47975,1000.);
#11085=VECTOR('',#47976,1000.);
#11086=VECTOR('',#47987,1000.);
#11087=VECTOR('',#47992,1000.);
#11088=VECTOR('',#47999,1000.);
#11089=VECTOR('',#48010,1000.);
#11090=VECTOR('',#48013,1000.);
#11091=VECTOR('',#48014,1000.);
#11092=VECTOR('',#48017,1000.);
#11093=VECTOR('',#48018,1000.);
#11094=VECTOR('',#48019,1000.);
#11095=VECTOR('',#48020,1000.);
#11096=VECTOR('',#48023,1000.);
#11097=VECTOR('',#48028,1000.);
#11098=VECTOR('',#48047,1000.);
#11099=VECTOR('',#48060,1000.);
#11100=VECTOR('',#48071,1000.);
#11101=VECTOR('',#48082,1000.);
#11102=VECTOR('',#48087,1000.);
#11103=VECTOR('',#48098,1000.);
#11104=VECTOR('',#48101,1000.);
#11105=VECTOR('',#48102,1000.);
#11106=VECTOR('',#48123,1000.);
#11107=VECTOR('',#48146,1000.);
#11108=VECTOR('',#48153,1000.);
#11109=VECTOR('',#48168,1000.);
#11110=VECTOR('',#48173,1000.);
#11111=VECTOR('',#48210,1000.);
#11112=VECTOR('',#48247,1000.);
#11113=VECTOR('',#48250,1000.);
#11114=VECTOR('',#48261,1000.);
#11115=VECTOR('',#48262,1000.);
#11116=VECTOR('',#48271,1000.);
#11117=VECTOR('',#48300,1000.);
#11118=VECTOR('',#48309,1000.);
#11119=VECTOR('',#48312,1000.);
#11120=VECTOR('',#48323,1000.);
#11121=VECTOR('',#48334,1000.);
#11122=VECTOR('',#48365,1000.);
#11123=VECTOR('',#48374,1000.);
#13335=CIRCLE('',#38090,13.016744254);
#13336=CIRCLE('',#38091,0.3);
#13337=CIRCLE('',#38092,13.316744254);
#13338=CIRCLE('',#38093,0.3);
#13339=CIRCLE('',#38095,25.7066723663);
#13340=CIRCLE('',#38096,25.7066723663);
#13341=CIRCLE('',#38098,0.300005627369098);
#13342=CIRCLE('',#38099,0.3);
#13343=CIRCLE('',#38101,12.2773059952);
#13344=CIRCLE('',#38102,12.2773059952);
#13345=CIRCLE('',#38104,25.2066723663);
#13346=CIRCLE('',#38105,0.5);
#13347=CIRCLE('',#38107,0.5);
#13348=CIRCLE('',#38108,11.7773059952);
#13349=CIRCLE('',#38110,25.2066723663);
#13350=CIRCLE('',#38111,4.5);
#13351=CIRCLE('',#38112,4.5);
#13352=CIRCLE('',#38113,11.7773059952);
#13353=CIRCLE('',#38115,5.);
#13354=CIRCLE('',#38116,0.5);
#13355=CIRCLE('',#38118,5.);
#13356=CIRCLE('',#38120,25.7066723663);
#13357=CIRCLE('',#38122,25.7066723663);
#13358=CIRCLE('',#38124,5.);
#13359=CIRCLE('',#38125,0.5);
#13360=CIRCLE('',#38127,5.);
#13361=CIRCLE('',#38129,0.300005627369097);
#13362=CIRCLE('',#38130,0.3);
#13363=CIRCLE('',#38132,12.2773059952);
#13364=CIRCLE('',#38134,12.2773059952);
#13365=CIRCLE('',#38136,13.616744254);
#13366=CIRCLE('',#38137,2.7);
#13367=CIRCLE('',#38138,15.3875296363);
#13368=CIRCLE('',#38140,0.3);
#13369=CIRCLE('',#38143,0.3);
#13370=CIRCLE('',#38144,13.316744254);
#13371=CIRCLE('',#38145,0.3);
#13372=CIRCLE('',#38147,0.3);
#13373=CIRCLE('',#38149,0.3);
#13374=CIRCLE('',#38151,13.316744254);
#13375=CIRCLE('',#38153,0.299999999999999);
#13376=CIRCLE('',#38155,0.3);
#13377=CIRCLE('',#38157,0.3);
#13378=CIRCLE('',#38160,13.616744254);
#13379=CIRCLE('',#38161,15.3875296363);
#13380=CIRCLE('',#38162,2.7);
#13381=CIRCLE('',#38164,0.3);
#13382=CIRCLE('',#38167,0.3);
#13383=CIRCLE('',#38168,0.3);
#13384=CIRCLE('',#38170,0.3);
#13385=CIRCLE('',#38172,13.316744254);
#13386=CIRCLE('',#38174,0.3);
#13387=CIRCLE('',#38176,0.300000000000001);
#13388=CIRCLE('',#38178,0.3);
#13389=CIRCLE('',#38180,0.3);
#13390=CIRCLE('',#38184,0.3);
#13391=CIRCLE('',#38186,13.7462109523);
#13392=CIRCLE('',#38187,2.8);
#13393=CIRCLE('',#38188,13.7462109523);
#13394=CIRCLE('',#38189,15.8875296363);
#13395=CIRCLE('',#38190,2.7);
#13396=CIRCLE('',#38191,15.8875296363);
#13397=CIRCLE('',#38193,0.3);
#13398=CIRCLE('',#38194,0.3);
#13399=CIRCLE('',#38196,0.3);
#13400=CIRCLE('',#38198,13.4462109523);
#13401=CIRCLE('',#38199,0.3);
#13402=CIRCLE('',#38201,13.4462109523);
#13403=CIRCLE('',#38203,2.5);
#13404=CIRCLE('',#38204,0.3);
#13405=CIRCLE('',#38206,2.5);
#13406=CIRCLE('',#38208,13.4462109523);
#13407=CIRCLE('',#38209,0.3);
#13408=CIRCLE('',#38211,13.4462109523);
#13409=CIRCLE('',#38213,0.3);
#13410=CIRCLE('',#38215,0.3);
#13411=CIRCLE('',#38217,0.3);
#13412=CIRCLE('',#38220,15.6875296363);
#13413=CIRCLE('',#38221,3.);
#13414=CIRCLE('',#38222,16.1875296363);
#13415=CIRCLE('',#38223,3.);
#13416=CIRCLE('',#38224,16.1875296363);
#13417=CIRCLE('',#38225,3.);
#13418=CIRCLE('',#38227,0.3);
#13419=CIRCLE('',#38228,0.300000000000001);
#13420=CIRCLE('',#38230,0.3);
#13421=CIRCLE('',#38231,0.6);
#13422=CIRCLE('',#38233,0.3);
#13423=CIRCLE('',#38234,13.016744254);
#13424=CIRCLE('',#38236,0.299999999999999);
#13425=CIRCLE('',#38237,0.6);
#13426=CIRCLE('',#38239,0.3);
#13427=CIRCLE('',#38241,0.3);
#13428=CIRCLE('',#38242,0.299999999999999);
#13429=CIRCLE('',#38244,0.6);
#13430=CIRCLE('',#38246,0.300000000000001);
#13431=CIRCLE('',#38247,0.6);
#13432=CIRCLE('',#38249,0.3);
#13433=CIRCLE('',#38251,0.3);
#13434=CIRCLE('',#38252,0.3);
#13435=CIRCLE('',#38254,0.3);
#13436=CIRCLE('',#38255,0.6);
#13437=CIRCLE('',#38257,0.3);
#13438=CIRCLE('',#38258,13.1462109523);
#13439=CIRCLE('',#38260,0.3);
#13440=CIRCLE('',#38261,2.2);
#13441=CIRCLE('',#38263,0.3);
#13442=CIRCLE('',#38264,13.1462109523);
#13443=CIRCLE('',#38266,0.3);
#13444=CIRCLE('',#38267,0.6);
#13445=CIRCLE('',#38269,0.3);
#13446=CIRCLE('',#38271,15.8875296363);
#13447=CIRCLE('',#38272,15.8875296363);
#13448=CIRCLE('',#38273,15.3875296363);
#13449=CIRCLE('',#38275,0.3);
#13450=CIRCLE('',#38276,0.3);
#13451=CIRCLE('',#38277,0.3);
#13452=CIRCLE('',#38279,0.299999999999999);
#13453=CIRCLE('',#38280,0.3);
#13454=CIRCLE('',#38281,0.299999999999998);
#13455=CIRCLE('',#38282,0.3);
#13456=CIRCLE('',#38284,16.1875296363);
#13457=CIRCLE('',#38285,0.3);
#13458=CIRCLE('',#38286,0.300000118306239);
#13459=CIRCLE('',#38291,16.1875296363);
#13460=CIRCLE('',#38292,0.3);
#13461=CIRCLE('',#38295,3.);
#13462=CIRCLE('',#38296,0.3);
#13463=CIRCLE('',#38299,0.3);
#13464=CIRCLE('',#38300,0.300000000000001);
#13465=CIRCLE('',#38301,0.3);
#13466=CIRCLE('',#38302,0.3);
#13467=CIRCLE('',#38304,0.3);
#13468=CIRCLE('',#38305,0.299999999999999);
#13469=CIRCLE('',#38306,0.299999999999999);
#13470=CIRCLE('',#38308,16.1875296363);
#13471=CIRCLE('',#38309,0.300000000015482);
#13472=CIRCLE('',#38310,0.3);
#13473=CIRCLE('',#38313,16.1875296363);
#13474=CIRCLE('',#38318,0.300000000000004);
#13475=CIRCLE('',#38319,0.3);
#13476=CIRCLE('',#38320,3.);
#13477=CIRCLE('',#38323,0.3);
#13478=CIRCLE('',#38325,3.);
#13479=CIRCLE('',#38328,0.3);
#13480=CIRCLE('',#38329,0.3);
#13481=CIRCLE('',#38330,0.299999999999999);
#13482=CIRCLE('',#38332,0.3);
#13483=CIRCLE('',#38333,0.299999999999998);
#13484=CIRCLE('',#38334,0.3);
#13485=CIRCLE('',#38335,0.3);
#13486=CIRCLE('',#38337,15.6875296363);
#13487=CIRCLE('',#38339,0.30000000000005);
#13488=CIRCLE('',#38340,15.6875296363);
#13489=CIRCLE('',#38344,15.6875296363);
#16291=VERTEX_POINT('',#95796);
#16292=VERTEX_POINT('',#95797);
#16293=VERTEX_POINT('',#95799);
#16294=VERTEX_POINT('',#95801);
#16295=VERTEX_POINT('',#95805);
#16296=VERTEX_POINT('',#95806);
#16297=VERTEX_POINT('',#95808);
#16298=VERTEX_POINT('',#95810);
#16299=VERTEX_POINT('',#95814);
#16300=VERTEX_POINT('',#95816);
#16301=VERTEX_POINT('',#95820);
#16302=VERTEX_POINT('',#95822);
#16303=VERTEX_POINT('',#95826);
#16304=VERTEX_POINT('',#95882);
#16305=VERTEX_POINT('',#95947);
#16306=VERTEX_POINT('',#95951);
#16307=VERTEX_POINT('',#95952);
#16308=VERTEX_POINT('',#95955);
#16309=VERTEX_POINT('',#95959);
#16310=VERTEX_POINT('',#95963);
#16311=VERTEX_POINT('',#95967);
#16312=VERTEX_POINT('',#95975);
#16313=VERTEX_POINT('',#95979);
#16314=VERTEX_POINT('',#95983);
#16315=VERTEX_POINT('',#95987);
#16316=VERTEX_POINT('',#95989);
#16317=VERTEX_POINT('',#96082);
#16318=VERTEX_POINT('',#96083);
#16319=VERTEX_POINT('',#96085);
#16320=VERTEX_POINT('',#96087);
#16321=VERTEX_POINT('',#96089);
#16322=VERTEX_POINT('',#96093);
#16323=VERTEX_POINT('',#96094);
#16324=VERTEX_POINT('',#96123);
#16325=VERTEX_POINT('',#96127);
#16326=VERTEX_POINT('',#96128);
#16327=VERTEX_POINT('',#96133);
#16328=VERTEX_POINT('',#96135);
#16329=VERTEX_POINT('',#96141);
#16330=VERTEX_POINT('',#96145);
#16331=VERTEX_POINT('',#96149);
#16332=VERTEX_POINT('',#96187);
#16333=VERTEX_POINT('',#96193);
#16334=VERTEX_POINT('',#96197);
#16335=VERTEX_POINT('',#96201);
#16336=VERTEX_POINT('',#96202);
#16337=VERTEX_POINT('',#96204);
#16338=VERTEX_POINT('',#96206);
#16339=VERTEX_POINT('',#96208);
#16340=VERTEX_POINT('',#96212);
#16341=VERTEX_POINT('',#96222);
#16342=VERTEX_POINT('',#96226);
#16343=VERTEX_POINT('',#96227);
#16344=VERTEX_POINT('',#96232);
#16345=VERTEX_POINT('',#96239);
#16346=VERTEX_POINT('',#96245);
#16347=VERTEX_POINT('',#96256);
#16348=VERTEX_POINT('',#96272);
#16349=VERTEX_POINT('',#96278);
#16350=VERTEX_POINT('',#96282);
#16351=VERTEX_POINT('',#96286);
#16352=VERTEX_POINT('',#96287);
#16353=VERTEX_POINT('',#96289);
#16354=VERTEX_POINT('',#96291);
#16355=VERTEX_POINT('',#96295);
#16356=VERTEX_POINT('',#96330);
#16357=VERTEX_POINT('',#96334);
#16358=VERTEX_POINT('',#96335);
#16359=VERTEX_POINT('',#96337);
#16360=VERTEX_POINT('',#96339);
#16361=VERTEX_POINT('',#96342);
#16362=VERTEX_POINT('',#96344);
#16363=VERTEX_POINT('',#96348);
#16364=VERTEX_POINT('',#96350);
#16365=VERTEX_POINT('',#96356);
#16366=VERTEX_POINT('',#96360);
#16367=VERTEX_POINT('',#96364);
#16368=VERTEX_POINT('',#96368);
#16369=VERTEX_POINT('',#96372);
#16370=VERTEX_POINT('',#96376);
#16371=VERTEX_POINT('',#96380);
#16372=VERTEX_POINT('',#96402);
#16373=VERTEX_POINT('',#96408);
#16374=VERTEX_POINT('',#96412);
#16375=VERTEX_POINT('',#96416);
#16376=VERTEX_POINT('',#96417);
#16377=VERTEX_POINT('',#96419);
#16378=VERTEX_POINT('',#96421);
#16379=VERTEX_POINT('',#96423);
#16380=VERTEX_POINT('',#96425);
#16381=VERTEX_POINT('',#96429);
#16382=VERTEX_POINT('',#96431);
#16383=VERTEX_POINT('',#96435);
#16384=VERTEX_POINT('',#96439);
#16385=VERTEX_POINT('',#96443);
#16386=VERTEX_POINT('',#96447);
#16387=VERTEX_POINT('',#96451);
#16388=VERTEX_POINT('',#96453);
#16389=VERTEX_POINT('',#96459);
#16390=VERTEX_POINT('',#96463);
#16391=VERTEX_POINT('',#96467);
#16392=VERTEX_POINT('',#96469);
#16393=VERTEX_POINT('',#96473);
#16394=VERTEX_POINT('',#96477);
#16395=VERTEX_POINT('',#96481);
#16396=VERTEX_POINT('',#96485);
#16397=VERTEX_POINT('',#96489);
#16398=VERTEX_POINT('',#96493);
#16399=VERTEX_POINT('',#96501);
#16400=VERTEX_POINT('',#96504);
#16401=VERTEX_POINT('',#96507);
#16402=VERTEX_POINT('',#96509);
#16403=VERTEX_POINT('',#96511);
#16404=VERTEX_POINT('',#96597);
#16405=VERTEX_POINT('',#96599);
#16406=VERTEX_POINT('',#96613);
#16407=VERTEX_POINT('',#96675);
#16408=VERTEX_POINT('',#96687);
#16409=VERTEX_POINT('',#96694);
#16410=VERTEX_POINT('',#96700);
#16411=VERTEX_POINT('',#96701);
#16412=VERTEX_POINT('',#96703);
#16413=VERTEX_POINT('',#96708);
#16414=VERTEX_POINT('',#96711);
#16415=VERTEX_POINT('',#96796);
#16416=VERTEX_POINT('',#96798);
#16417=VERTEX_POINT('',#96837);
#16418=VERTEX_POINT('',#96894);
#16419=VERTEX_POINT('',#96946);
#16420=VERTEX_POINT('',#96948);
#16421=VERTEX_POINT('',#97003);
#16422=VERTEX_POINT('',#97005);
#16423=VERTEX_POINT('',#97060);
#16424=VERTEX_POINT('',#97063);
#16425=VERTEX_POINT('',#97066);
#16426=VERTEX_POINT('',#97067);
#16427=VERTEX_POINT('',#97069);
#16428=VERTEX_POINT('',#97076);
#16429=VERTEX_POINT('',#97133);
#16430=VERTEX_POINT('',#97183);
#16431=VERTEX_POINT('',#97240);
#21192=EDGE_CURVE('',#16291,#16292,#13335,.T.);
#21193=EDGE_CURVE('',#16291,#16293,#13336,.T.);
#21194=EDGE_CURVE('',#16293,#16294,#13337,.T.);
#21195=EDGE_CURVE('',#16292,#16294,#13338,.T.);
#21196=EDGE_CURVE('',#16295,#16296,#13339,.T.);
#21197=EDGE_CURVE('',#16297,#16295,#9220,.T.);
#21198=EDGE_CURVE('',#16298,#16297,#13340,.T.);
#21199=EDGE_CURVE('',#16298,#16296,#9221,.T.);
#21200=EDGE_CURVE('',#16299,#16296,#13341,.T.);
#21201=EDGE_CURVE('',#16300,#16298,#13342,.T.);
#21202=EDGE_CURVE('',#16300,#16299,#9222,.T.);
#21203=EDGE_CURVE('',#16299,#16301,#13343,.T.);
#21204=EDGE_CURVE('',#16302,#16300,#13344,.T.);
#21205=EDGE_CURVE('',#16302,#16301,#9223,.T.);
#21206=EDGE_CURVE('',#16296,#16303,#2003,.T.);
#21207=EDGE_CURVE('',#16304,#16303,#13345,.T.);
#21208=EDGE_CURVE('',#16295,#16304,#13346,.T.);
#21209=EDGE_CURVE('',#16299,#16303,#2004,.T.);
#21210=EDGE_CURVE('',#16301,#16305,#13347,.T.);
#21211=EDGE_CURVE('',#16303,#16305,#13348,.T.);
#21212=EDGE_CURVE('',#16306,#16307,#13349,.T.);
#21213=EDGE_CURVE('',#16307,#16304,#13350,.T.);
#21214=EDGE_CURVE('',#16305,#16308,#13351,.T.);
#21215=EDGE_CURVE('',#16308,#16306,#13352,.T.);
#21216=EDGE_CURVE('',#16309,#16295,#13353,.T.);
#21217=EDGE_CURVE('',#16309,#16307,#13354,.T.);
#21218=EDGE_CURVE('',#16310,#16309,#9224,.T.);
#21219=EDGE_CURVE('',#16297,#16310,#13355,.T.);
#21220=EDGE_CURVE('',#16311,#16306,#2005,.T.);
#21221=EDGE_CURVE('',#16311,#16309,#13356,.T.);
#21222=EDGE_CURVE('',#16312,#16311,#9225,.T.);
#21223=EDGE_CURVE('',#16312,#16310,#13357,.T.);
#21224=EDGE_CURVE('',#16301,#16313,#13358,.T.);
#21225=EDGE_CURVE('',#16313,#16308,#13359,.T.);
#21226=EDGE_CURVE('',#16314,#16302,#13360,.T.);
#21227=EDGE_CURVE('',#16314,#16313,#9226,.T.);
#21228=EDGE_CURVE('',#16311,#16315,#13361,.T.);
#21229=EDGE_CURVE('',#16316,#16315,#9227,.T.);
#21230=EDGE_CURVE('',#16312,#16316,#13362,.T.);
#21231=EDGE_CURVE('',#16315,#16306,#2006,.T.);
#21232=EDGE_CURVE('',#16313,#16315,#13363,.T.);
#21233=EDGE_CURVE('',#16314,#16316,#13364,.T.);
#21234=EDGE_CURVE('',#16317,#16318,#9228,.T.);
#21235=EDGE_CURVE('',#16319,#16317,#13365,.T.);
#21236=EDGE_CURVE('',#16320,#16319,#9229,.T.);
#21237=EDGE_CURVE('',#16321,#16320,#13366,.T.);
#21238=EDGE_CURVE('',#16318,#16321,#13367,.T.);
#21239=EDGE_CURVE('',#16322,#16323,#2007,.T.);
#21240=EDGE_CURVE('',#16320,#16322,#2008,.T.);
#21241=EDGE_CURVE('',#16319,#16324,#13368,.T.);
#21242=EDGE_CURVE('',#16323,#16324,#9230,.T.);
#21243=EDGE_CURVE('',#16325,#16326,#9231,.T.);
#21244=EDGE_CURVE('',#16323,#16325,#9232,.T.);
#21245=EDGE_CURVE('',#16326,#16324,#9233,.T.);
#21246=EDGE_CURVE('',#16317,#16327,#13369,.T.);
#21247=EDGE_CURVE('',#16328,#16327,#13370,.T.);
#21248=EDGE_CURVE('',#16319,#16328,#13371,.T.);
#21249=EDGE_CURVE('',#16324,#16328,#13372,.T.);
#21250=EDGE_CURVE('',#16326,#16329,#13373,.T.);
#21251=EDGE_CURVE('',#16329,#16328,#9234,.T.);
#21252=EDGE_CURVE('',#16330,#16327,#9235,.T.);
#21253=EDGE_CURVE('',#16329,#16330,#13374,.T.);
#21254=EDGE_CURVE('',#16331,#16318,#2009,.T.);
#21255=EDGE_CURVE('',#16332,#16331,#9236,.T.);
#21256=EDGE_CURVE('',#16317,#16332,#13375,.T.);
#21257=EDGE_CURVE('',#16327,#16332,#13376,.T.);
#21258=EDGE_CURVE('',#16330,#16333,#13377,.T.);
#21259=EDGE_CURVE('',#16333,#16332,#9237,.T.);
#21260=EDGE_CURVE('',#16334,#16331,#9238,.T.);
#21261=EDGE_CURVE('',#16333,#16334,#9239,.T.);
#21262=EDGE_CURVE('',#16335,#16336,#9240,.T.);
#21263=EDGE_CURVE('',#16337,#16335,#13378,.T.);
#21264=EDGE_CURVE('',#16338,#16337,#9241,.T.);
#21265=EDGE_CURVE('',#16339,#16338,#13379,.T.);
#21266=EDGE_CURVE('',#16336,#16339,#13380,.T.);
#21267=EDGE_CURVE('',#16338,#16340,#2010,.T.);
#21268=EDGE_CURVE('',#16337,#16341,#13381,.T.);
#21269=EDGE_CURVE('',#16340,#16341,#9242,.T.);
#21270=EDGE_CURVE('',#16342,#16343,#9243,.T.);
#21271=EDGE_CURVE('',#16340,#16342,#9244,.T.);
#21272=EDGE_CURVE('',#16341,#16343,#9245,.T.);
#21273=EDGE_CURVE('',#16337,#16344,#13382,.T.);
#21274=EDGE_CURVE('',#16341,#16344,#13383,.T.);
#21275=EDGE_CURVE('',#16343,#16293,#13384,.T.);
#21276=EDGE_CURVE('',#16344,#16293,#9246,.T.);
#21277=EDGE_CURVE('',#16344,#16345,#13385,.T.);
#21278=EDGE_CURVE('',#16294,#16345,#9247,.T.);
#21279=EDGE_CURVE('',#16335,#16345,#13386,.T.);
#21280=EDGE_CURVE('',#16346,#16336,#2011,.T.);
#21281=EDGE_CURVE('',#16347,#16346,#2012,.T.);
#21282=EDGE_CURVE('',#16348,#16347,#9248,.T.);
#21283=EDGE_CURVE('',#16335,#16348,#13387,.T.);
#21284=EDGE_CURVE('',#16345,#16348,#13388,.T.);
#21285=EDGE_CURVE('',#16294,#16349,#13389,.T.);
#21286=EDGE_CURVE('',#16349,#16348,#9249,.T.);
#21287=EDGE_CURVE('',#16350,#16347,#9250,.T.);
#21288=EDGE_CURVE('',#16349,#16350,#9251,.T.);
#21289=EDGE_CURVE('',#16351,#16352,#9252,.T.);
#21290=EDGE_CURVE('',#16352,#16353,#9253,.T.);
#21291=EDGE_CURVE('',#16354,#16353,#9254,.T.);
#21292=EDGE_CURVE('',#16354,#16351,#9255,.T.);
#21293=EDGE_CURVE('',#16353,#16355,#2013,.T.);
#21294=EDGE_CURVE('',#16356,#16355,#9256,.T.);
#21295=EDGE_CURVE('',#16354,#16356,#13390,.T.);
#21296=EDGE_CURVE('',#16357,#16358,#9257,.T.);
#21297=EDGE_CURVE('',#16358,#16359,#13391,.T.);
#21298=EDGE_CURVE('',#16359,#16360,#13392,.T.);
#21299=EDGE_CURVE('',#16360,#16356,#13393,.T.);
#21300=EDGE_CURVE('',#16355,#16361,#13394,.T.);
#21301=EDGE_CURVE('',#16361,#16362,#13395,.T.);
#21302=EDGE_CURVE('',#16362,#16357,#13396,.T.);
#21303=EDGE_CURVE('',#16363,#16351,#13397,.T.);
#21304=EDGE_CURVE('',#16364,#16354,#13398,.T.);
#21305=EDGE_CURVE('',#16364,#16363,#9258,.T.);
#21306=EDGE_CURVE('',#16364,#16356,#13399,.T.);
#21307=EDGE_CURVE('',#16365,#16364,#13400,.T.);
#21308=EDGE_CURVE('',#16365,#16360,#13401,.T.);
#21309=EDGE_CURVE('',#16365,#16366,#9259,.T.);
#21310=EDGE_CURVE('',#16366,#16363,#13402,.T.);
#21311=EDGE_CURVE('',#16367,#16365,#13403,.T.);
#21312=EDGE_CURVE('',#16367,#16359,#13404,.T.);
#21313=EDGE_CURVE('',#16367,#16368,#9260,.T.);
#21314=EDGE_CURVE('',#16368,#16366,#13405,.T.);
#21315=EDGE_CURVE('',#16369,#16367,#13406,.T.);
#21316=EDGE_CURVE('',#16369,#16358,#13407,.T.);
#21317=EDGE_CURVE('',#16370,#16369,#9261,.T.);
#21318=EDGE_CURVE('',#16370,#16368,#13408,.T.);
#21319=EDGE_CURVE('',#16357,#16371,#2014,.T.);
#21320=EDGE_CURVE('',#16371,#16372,#9262,.T.);
#21321=EDGE_CURVE('',#16372,#16358,#13409,.T.);
#21322=EDGE_CURVE('',#16372,#16369,#13410,.T.);
#21323=EDGE_CURVE('',#16373,#16370,#13411,.T.);
#21324=EDGE_CURVE('',#16373,#16372,#9263,.T.);
#21325=EDGE_CURVE('',#16371,#16374,#9264,.T.);
#21326=EDGE_CURVE('',#16374,#16373,#9265,.T.);
#21327=EDGE_CURVE('',#16375,#16376,#13412,.T.);
#21328=EDGE_CURVE('',#16377,#16376,#13413,.T.);
#21329=EDGE_CURVE('',#16377,#16378,#13414,.T.);
#21330=EDGE_CURVE('',#16379,#16378,#13415,.T.);
#21331=EDGE_CURVE('',#16379,#16380,#13416,.T.);
#21332=EDGE_CURVE('',#16375,#16380,#13417,.T.);
#21333=EDGE_CURVE('',#16381,#16325,#13418,.T.);
#21334=EDGE_CURVE('',#16382,#16326,#13419,.T.);
#21335=EDGE_CURVE('',#16381,#16382,#9266,.T.);
#21336=EDGE_CURVE('',#16383,#16329,#13420,.T.);
#21337=EDGE_CURVE('',#16382,#16383,#13421,.T.);
#21338=EDGE_CURVE('',#16384,#16330,#13422,.T.);
#21339=EDGE_CURVE('',#16383,#16384,#13423,.T.);
#21340=EDGE_CURVE('',#16385,#16333,#13424,.T.);
#21341=EDGE_CURVE('',#16384,#16385,#13425,.T.);
#21342=EDGE_CURVE('',#16386,#16334,#13426,.T.);
#21343=EDGE_CURVE('',#16385,#16386,#9267,.T.);
#21344=EDGE_CURVE('',#16387,#16342,#13427,.T.);
#21345=EDGE_CURVE('',#16388,#16343,#13428,.T.);
#21346=EDGE_CURVE('',#16387,#16388,#9268,.T.);
#21347=EDGE_CURVE('',#16388,#16291,#13429,.T.);
#21348=EDGE_CURVE('',#16389,#16349,#13430,.T.);
#21349=EDGE_CURVE('',#16292,#16389,#13431,.T.);
#21350=EDGE_CURVE('',#16390,#16350,#13432,.T.);
#21351=EDGE_CURVE('',#16389,#16390,#9269,.T.);
#21352=EDGE_CURVE('',#16351,#16391,#13433,.T.);
#21353=EDGE_CURVE('',#16391,#16392,#9270,.T.);
#21354=EDGE_CURVE('',#16352,#16392,#13434,.T.);
#21355=EDGE_CURVE('',#16363,#16393,#13435,.T.);
#21356=EDGE_CURVE('',#16393,#16391,#13436,.T.);
#21357=EDGE_CURVE('',#16366,#16394,#13437,.T.);
#21358=EDGE_CURVE('',#16394,#16393,#13438,.T.);
#21359=EDGE_CURVE('',#16368,#16395,#13439,.T.);
#21360=EDGE_CURVE('',#16395,#16394,#13440,.T.);
#21361=EDGE_CURVE('',#16370,#16396,#13441,.T.);
#21362=EDGE_CURVE('',#16396,#16395,#13442,.T.);
#21363=EDGE_CURVE('',#16373,#16397,#13443,.T.);
#21364=EDGE_CURVE('',#16397,#16396,#13444,.T.);
#21365=EDGE_CURVE('',#16374,#16398,#13445,.T.);
#21366=EDGE_CURVE('',#16398,#16397,#9271,.T.);
#21367=EDGE_CURVE('',#16392,#16390,#13446,.T.);
#21368=EDGE_CURVE('',#16381,#16398,#13447,.T.);
#21369=EDGE_CURVE('',#16387,#16386,#13448,.T.);
#21370=EDGE_CURVE('',#16399,#16350,#13449,.T.);
#21371=EDGE_CURVE('',#16390,#16399,#13450,.T.);
#21372=EDGE_CURVE('',#16400,#16390,#13451,.T.);
#21373=EDGE_CURVE('',#16392,#16401,#13452,.T.);
#21374=EDGE_CURVE('',#16402,#16401,#13453,.T.);
#21375=EDGE_CURVE('',#16403,#16402,#13454,.T.);
#21376=EDGE_CURVE('',#16352,#16402,#13455,.T.);
#21377=EDGE_CURVE('',#16401,#16399,#13456,.T.);
#21378=EDGE_CURVE('',#16404,#16347,#13457,.T.);
#21379=EDGE_CURVE('',#16405,#16346,#13458,.T.);
#21380=EDGE_CURVE('',#16404,#16405,#2015,.T.);
#21381=EDGE_CURVE('',#16399,#16404,#9272,.T.);
#21382=EDGE_CURVE('',#16401,#16406,#9273,.T.);
#21383=EDGE_CURVE('',#16353,#16406,#2016,.T.);
#21384=EDGE_CURVE('',#16406,#16407,#2017,.T.);
#21385=EDGE_CURVE('',#16355,#16407,#706,.T.);
#21386=EDGE_CURVE('',#16407,#16408,#13459,.T.);
#21387=EDGE_CURVE('',#16361,#16408,#13460,.T.);
#21388=EDGE_CURVE('',#16405,#16380,#9274,.T.);
#21389=EDGE_CURVE('',#16408,#16379,#9275,.T.);
#21390=EDGE_CURVE('',#16408,#16409,#13461,.T.);
#21391=EDGE_CURVE('',#16362,#16409,#13462,.T.);
#21392=EDGE_CURVE('',#16409,#16378,#9276,.T.);
#21393=EDGE_CURVE('',#16410,#16411,#13463,.T.);
#21394=EDGE_CURVE('',#16412,#16411,#13464,.T.);
#21395=EDGE_CURVE('',#16411,#16325,#13465,.T.);
#21396=EDGE_CURVE('',#16410,#16381,#13466,.T.);
#21397=EDGE_CURVE('',#16374,#16413,#13467,.T.);
#21398=EDGE_CURVE('',#16413,#16398,#13468,.T.);
#21399=EDGE_CURVE('',#16414,#16398,#13469,.T.);
#21400=EDGE_CURVE('',#16410,#16413,#13470,.T.);
#21401=EDGE_CURVE('',#16415,#16322,#13471,.T.);
#21402=EDGE_CURVE('',#16416,#16323,#13472,.T.);
#21403=EDGE_CURVE('',#16415,#16416,#2018,.T.);
#21404=EDGE_CURVE('',#16416,#16410,#9277,.T.);
#21405=EDGE_CURVE('',#16409,#16417,#13473,.T.);
#21406=EDGE_CURVE('',#16357,#16417,#707,.T.);
#21407=EDGE_CURVE('',#16417,#16418,#2019,.T.);
#21408=EDGE_CURVE('',#16371,#16418,#2020,.T.);
#21409=EDGE_CURVE('',#16418,#16413,#9278,.T.);
#21410=EDGE_CURVE('',#16415,#16377,#9279,.T.);
#21411=EDGE_CURVE('',#16419,#16336,#13474,.T.);
#21412=EDGE_CURVE('',#16420,#16339,#13475,.T.);
#21413=EDGE_CURVE('',#16419,#16420,#13476,.T.);
#21414=EDGE_CURVE('',#16405,#16419,#2021,.T.);
#21415=EDGE_CURVE('',#16420,#16375,#9280,.T.);
#21416=EDGE_CURVE('',#16421,#16321,#13477,.T.);
#21417=EDGE_CURVE('',#16422,#16320,#708,.T.);
#21418=EDGE_CURVE('',#16421,#16422,#13478,.T.);
#21419=EDGE_CURVE('',#16422,#16415,#2022,.T.);
#21420=EDGE_CURVE('',#16421,#16376,#9281,.T.);
#21421=EDGE_CURVE('',#16423,#16334,#13479,.T.);
#21422=EDGE_CURVE('',#16386,#16423,#13480,.T.);
#21423=EDGE_CURVE('',#16424,#16386,#13481,.T.);
#21424=EDGE_CURVE('',#16425,#16426,#13482,.T.);
#21425=EDGE_CURVE('',#16427,#16426,#13483,.T.);
#21426=EDGE_CURVE('',#16426,#16342,#13484,.T.);
#21427=EDGE_CURVE('',#16425,#16387,#13485,.T.);
#21428=EDGE_CURVE('',#16425,#16423,#13486,.T.);
#21429=EDGE_CURVE('',#16428,#16318,#13487,.T.);
#21430=EDGE_CURVE('',#16428,#16421,#13488,.T.);
#21431=EDGE_CURVE('',#16429,#16331,#2023,.T.);
#21432=EDGE_CURVE('',#16429,#16428,#2024,.T.);
#21433=EDGE_CURVE('',#16423,#16429,#9282,.T.);
#21434=EDGE_CURVE('',#16430,#16338,#709,.T.);
#21435=EDGE_CURVE('',#16420,#16430,#13489,.T.);
#21436=EDGE_CURVE('',#16431,#16340,#2025,.T.);
#21437=EDGE_CURVE('',#16430,#16431,#2026,.T.);
#21438=EDGE_CURVE('',#16431,#16425,#9283,.T.);
#30841=ORIENTED_EDGE('',*,*,#21192,.F.);
#30842=ORIENTED_EDGE('',*,*,#21193,.T.);
#30843=ORIENTED_EDGE('',*,*,#21194,.T.);
#30844=ORIENTED_EDGE('',*,*,#21195,.F.);
#30845=ORIENTED_EDGE('',*,*,#21196,.F.);
#30846=ORIENTED_EDGE('',*,*,#21197,.F.);
#30847=ORIENTED_EDGE('',*,*,#21198,.F.);
#30848=ORIENTED_EDGE('',*,*,#21199,.T.);
#30849=ORIENTED_EDGE('',*,*,#21200,.T.);
#30850=ORIENTED_EDGE('',*,*,#21199,.F.);
#30851=ORIENTED_EDGE('',*,*,#21201,.F.);
#30852=ORIENTED_EDGE('',*,*,#21202,.T.);
#30853=ORIENTED_EDGE('',*,*,#21203,.F.);
#30854=ORIENTED_EDGE('',*,*,#21202,.F.);
#30855=ORIENTED_EDGE('',*,*,#21204,.F.);
#30856=ORIENTED_EDGE('',*,*,#21205,.T.);
#30857=ORIENTED_EDGE('',*,*,#21206,.T.);
#30858=ORIENTED_EDGE('',*,*,#21207,.F.);
#30859=ORIENTED_EDGE('',*,*,#21208,.F.);
#30860=ORIENTED_EDGE('',*,*,#21196,.T.);
#30861=ORIENTED_EDGE('',*,*,#21209,.T.);
#30862=ORIENTED_EDGE('',*,*,#21206,.F.);
#30863=ORIENTED_EDGE('',*,*,#21200,.F.);
#30864=ORIENTED_EDGE('',*,*,#21209,.F.);
#30865=ORIENTED_EDGE('',*,*,#21203,.T.);
#30866=ORIENTED_EDGE('',*,*,#21210,.T.);
#30867=ORIENTED_EDGE('',*,*,#21211,.F.);
#30868=ORIENTED_EDGE('',*,*,#21212,.T.);
#30869=ORIENTED_EDGE('',*,*,#21213,.T.);
#30870=ORIENTED_EDGE('',*,*,#21207,.T.);
#30871=ORIENTED_EDGE('',*,*,#21211,.T.);
#30872=ORIENTED_EDGE('',*,*,#21214,.T.);
#30873=ORIENTED_EDGE('',*,*,#21215,.T.);
#30874=ORIENTED_EDGE('',*,*,#21216,.T.);
#30875=ORIENTED_EDGE('',*,*,#21208,.T.);
#30876=ORIENTED_EDGE('',*,*,#21213,.F.);
#30877=ORIENTED_EDGE('',*,*,#21217,.F.);
#30878=ORIENTED_EDGE('',*,*,#21216,.F.);
#30879=ORIENTED_EDGE('',*,*,#21218,.F.);
#30880=ORIENTED_EDGE('',*,*,#21219,.F.);
#30881=ORIENTED_EDGE('',*,*,#21197,.T.);
#30882=ORIENTED_EDGE('',*,*,#21220,.F.);
#30883=ORIENTED_EDGE('',*,*,#21221,.T.);
#30884=ORIENTED_EDGE('',*,*,#21217,.T.);
#30885=ORIENTED_EDGE('',*,*,#21212,.F.);
#30886=ORIENTED_EDGE('',*,*,#21221,.F.);
#30887=ORIENTED_EDGE('',*,*,#21222,.F.);
#30888=ORIENTED_EDGE('',*,*,#21223,.T.);
#30889=ORIENTED_EDGE('',*,*,#21218,.T.);
#30890=ORIENTED_EDGE('',*,*,#21224,.T.);
#30891=ORIENTED_EDGE('',*,*,#21225,.T.);
#30892=ORIENTED_EDGE('',*,*,#21214,.F.);
#30893=ORIENTED_EDGE('',*,*,#21210,.F.);
#30894=ORIENTED_EDGE('',*,*,#21224,.F.);
#30895=ORIENTED_EDGE('',*,*,#21205,.F.);
#30896=ORIENTED_EDGE('',*,*,#21226,.F.);
#30897=ORIENTED_EDGE('',*,*,#21227,.T.);
#30898=ORIENTED_EDGE('',*,*,#21228,.T.);
#30899=ORIENTED_EDGE('',*,*,#21229,.F.);
#30900=ORIENTED_EDGE('',*,*,#21230,.F.);
#30901=ORIENTED_EDGE('',*,*,#21222,.T.);
#30902=ORIENTED_EDGE('',*,*,#21231,.T.);
#30903=ORIENTED_EDGE('',*,*,#21215,.F.);
#30904=ORIENTED_EDGE('',*,*,#21225,.F.);
#30905=ORIENTED_EDGE('',*,*,#21232,.T.);
#30906=ORIENTED_EDGE('',*,*,#21220,.T.);
#30907=ORIENTED_EDGE('',*,*,#21231,.F.);
#30908=ORIENTED_EDGE('',*,*,#21228,.F.);
#30909=ORIENTED_EDGE('',*,*,#21232,.F.);
#30910=ORIENTED_EDGE('',*,*,#21227,.F.);
#30911=ORIENTED_EDGE('',*,*,#21233,.T.);
#30912=ORIENTED_EDGE('',*,*,#21229,.T.);
#30913=ORIENTED_EDGE('',*,*,#21234,.F.);
#30914=ORIENTED_EDGE('',*,*,#21235,.F.);
#30915=ORIENTED_EDGE('',*,*,#21236,.F.);
#30916=ORIENTED_EDGE('',*,*,#21237,.F.);
#30917=ORIENTED_EDGE('',*,*,#21238,.F.);
#30918=ORIENTED_EDGE('',*,*,#21239,.F.);
#30919=ORIENTED_EDGE('',*,*,#21240,.F.);
#30920=ORIENTED_EDGE('',*,*,#21236,.T.);
#30921=ORIENTED_EDGE('',*,*,#21241,.T.);
#30922=ORIENTED_EDGE('',*,*,#21242,.F.);
#30923=ORIENTED_EDGE('',*,*,#21243,.F.);
#30924=ORIENTED_EDGE('',*,*,#21244,.F.);
#30925=ORIENTED_EDGE('',*,*,#21242,.T.);
#30926=ORIENTED_EDGE('',*,*,#21245,.F.);
#30927=ORIENTED_EDGE('',*,*,#21235,.T.);
#30928=ORIENTED_EDGE('',*,*,#21246,.T.);
#30929=ORIENTED_EDGE('',*,*,#21247,.F.);
#30930=ORIENTED_EDGE('',*,*,#21248,.F.);
#30931=ORIENTED_EDGE('',*,*,#21248,.T.);
#30932=ORIENTED_EDGE('',*,*,#21249,.F.);
#30933=ORIENTED_EDGE('',*,*,#21241,.F.);
#30934=ORIENTED_EDGE('',*,*,#21250,.F.);
#30935=ORIENTED_EDGE('',*,*,#21245,.T.);
#30936=ORIENTED_EDGE('',*,*,#21249,.T.);
#30937=ORIENTED_EDGE('',*,*,#21251,.F.);
#30938=ORIENTED_EDGE('',*,*,#21251,.T.);
#30939=ORIENTED_EDGE('',*,*,#21247,.T.);
#30940=ORIENTED_EDGE('',*,*,#21252,.F.);
#30941=ORIENTED_EDGE('',*,*,#21253,.F.);
#30942=ORIENTED_EDGE('',*,*,#21254,.F.);
#30943=ORIENTED_EDGE('',*,*,#21255,.F.);
#30944=ORIENTED_EDGE('',*,*,#21256,.F.);
#30945=ORIENTED_EDGE('',*,*,#21234,.T.);
#30946=ORIENTED_EDGE('',*,*,#21256,.T.);
#30947=ORIENTED_EDGE('',*,*,#21257,.F.);
#30948=ORIENTED_EDGE('',*,*,#21246,.F.);
#30949=ORIENTED_EDGE('',*,*,#21258,.F.);
#30950=ORIENTED_EDGE('',*,*,#21252,.T.);
#30951=ORIENTED_EDGE('',*,*,#21257,.T.);
#30952=ORIENTED_EDGE('',*,*,#21259,.F.);
#30953=ORIENTED_EDGE('',*,*,#21259,.T.);
#30954=ORIENTED_EDGE('',*,*,#21255,.T.);
#30955=ORIENTED_EDGE('',*,*,#21260,.F.);
#30956=ORIENTED_EDGE('',*,*,#21261,.F.);
#30957=ORIENTED_EDGE('',*,*,#21262,.F.);
#30958=ORIENTED_EDGE('',*,*,#21263,.F.);
#30959=ORIENTED_EDGE('',*,*,#21264,.F.);
#30960=ORIENTED_EDGE('',*,*,#21265,.F.);
#30961=ORIENTED_EDGE('',*,*,#21266,.F.);
#30962=ORIENTED_EDGE('',*,*,#21267,.F.);
#30963=ORIENTED_EDGE('',*,*,#21264,.T.);
#30964=ORIENTED_EDGE('',*,*,#21268,.T.);
#30965=ORIENTED_EDGE('',*,*,#21269,.F.);
#30966=ORIENTED_EDGE('',*,*,#21270,.F.);
#30967=ORIENTED_EDGE('',*,*,#21271,.F.);
#30968=ORIENTED_EDGE('',*,*,#21269,.T.);
#30969=ORIENTED_EDGE('',*,*,#21272,.T.);
#30970=ORIENTED_EDGE('',*,*,#21273,.T.);
#30971=ORIENTED_EDGE('',*,*,#21274,.F.);
#30972=ORIENTED_EDGE('',*,*,#21268,.F.);
#30973=ORIENTED_EDGE('',*,*,#21275,.F.);
#30974=ORIENTED_EDGE('',*,*,#21272,.F.);
#30975=ORIENTED_EDGE('',*,*,#21274,.T.);
#30976=ORIENTED_EDGE('',*,*,#21276,.T.);
#30977=ORIENTED_EDGE('',*,*,#21276,.F.);
#30978=ORIENTED_EDGE('',*,*,#21277,.T.);
#30979=ORIENTED_EDGE('',*,*,#21278,.F.);
#30980=ORIENTED_EDGE('',*,*,#21194,.F.);
#30981=ORIENTED_EDGE('',*,*,#21263,.T.);
#30982=ORIENTED_EDGE('',*,*,#21279,.T.);
#30983=ORIENTED_EDGE('',*,*,#21277,.F.);
#30984=ORIENTED_EDGE('',*,*,#21273,.F.);
#30985=ORIENTED_EDGE('',*,*,#21280,.F.);
#30986=ORIENTED_EDGE('',*,*,#21281,.F.);
#30987=ORIENTED_EDGE('',*,*,#21282,.F.);
#30988=ORIENTED_EDGE('',*,*,#21283,.F.);
#30989=ORIENTED_EDGE('',*,*,#21262,.T.);
#30990=ORIENTED_EDGE('',*,*,#21283,.T.);
#30991=ORIENTED_EDGE('',*,*,#21284,.F.);
#30992=ORIENTED_EDGE('',*,*,#21279,.F.);
#30993=ORIENTED_EDGE('',*,*,#21285,.F.);
#30994=ORIENTED_EDGE('',*,*,#21278,.T.);
#30995=ORIENTED_EDGE('',*,*,#21284,.T.);
#30996=ORIENTED_EDGE('',*,*,#21286,.F.);
#30997=ORIENTED_EDGE('',*,*,#21286,.T.);
#30998=ORIENTED_EDGE('',*,*,#21282,.T.);
#30999=ORIENTED_EDGE('',*,*,#21287,.F.);
#31000=ORIENTED_EDGE('',*,*,#21288,.F.);
#31001=ORIENTED_EDGE('',*,*,#21289,.T.);
#31002=ORIENTED_EDGE('',*,*,#21290,.T.);
#31003=ORIENTED_EDGE('',*,*,#21291,.F.);
#31004=ORIENTED_EDGE('',*,*,#21292,.T.);
#31005=ORIENTED_EDGE('',*,*,#21293,.T.);
#31006=ORIENTED_EDGE('',*,*,#21294,.F.);
#31007=ORIENTED_EDGE('',*,*,#21295,.F.);
#31008=ORIENTED_EDGE('',*,*,#21291,.T.);
#31009=ORIENTED_EDGE('',*,*,#21296,.T.);
#31010=ORIENTED_EDGE('',*,*,#21297,.T.);
#31011=ORIENTED_EDGE('',*,*,#21298,.T.);
#31012=ORIENTED_EDGE('',*,*,#21299,.T.);
#31013=ORIENTED_EDGE('',*,*,#21294,.T.);
#31014=ORIENTED_EDGE('',*,*,#21300,.T.);
#31015=ORIENTED_EDGE('',*,*,#21301,.T.);
#31016=ORIENTED_EDGE('',*,*,#21302,.T.);
#31017=ORIENTED_EDGE('',*,*,#21303,.T.);
#31018=ORIENTED_EDGE('',*,*,#21292,.F.);
#31019=ORIENTED_EDGE('',*,*,#21304,.F.);
#31020=ORIENTED_EDGE('',*,*,#21305,.T.);
#31021=ORIENTED_EDGE('',*,*,#21304,.T.);
#31022=ORIENTED_EDGE('',*,*,#21295,.T.);
#31023=ORIENTED_EDGE('',*,*,#21306,.F.);
#31024=ORIENTED_EDGE('',*,*,#21307,.T.);
#31025=ORIENTED_EDGE('',*,*,#21306,.T.);
#31026=ORIENTED_EDGE('',*,*,#21299,.F.);
#31027=ORIENTED_EDGE('',*,*,#21308,.F.);
#31028=ORIENTED_EDGE('',*,*,#21305,.F.);
#31029=ORIENTED_EDGE('',*,*,#21307,.F.);
#31030=ORIENTED_EDGE('',*,*,#21309,.T.);
#31031=ORIENTED_EDGE('',*,*,#21310,.T.);
#31032=ORIENTED_EDGE('',*,*,#21311,.T.);
#31033=ORIENTED_EDGE('',*,*,#21308,.T.);
#31034=ORIENTED_EDGE('',*,*,#21298,.F.);
#31035=ORIENTED_EDGE('',*,*,#21312,.F.);
#31036=ORIENTED_EDGE('',*,*,#21309,.F.);
#31037=ORIENTED_EDGE('',*,*,#21311,.F.);
#31038=ORIENTED_EDGE('',*,*,#21313,.T.);
#31039=ORIENTED_EDGE('',*,*,#21314,.T.);
#31040=ORIENTED_EDGE('',*,*,#21315,.T.);
#31041=ORIENTED_EDGE('',*,*,#21312,.T.);
#31042=ORIENTED_EDGE('',*,*,#21297,.F.);
#31043=ORIENTED_EDGE('',*,*,#21316,.F.);
#31044=ORIENTED_EDGE('',*,*,#21313,.F.);
#31045=ORIENTED_EDGE('',*,*,#21315,.F.);
#31046=ORIENTED_EDGE('',*,*,#21317,.F.);
#31047=ORIENTED_EDGE('',*,*,#21318,.T.);
#31048=ORIENTED_EDGE('',*,*,#21319,.T.);
#31049=ORIENTED_EDGE('',*,*,#21320,.T.);
#31050=ORIENTED_EDGE('',*,*,#21321,.T.);
#31051=ORIENTED_EDGE('',*,*,#21296,.F.);
#31052=ORIENTED_EDGE('',*,*,#21322,.T.);
#31053=ORIENTED_EDGE('',*,*,#21316,.T.);
#31054=ORIENTED_EDGE('',*,*,#21321,.F.);
#31055=ORIENTED_EDGE('',*,*,#21323,.T.);
#31056=ORIENTED_EDGE('',*,*,#21317,.T.);
#31057=ORIENTED_EDGE('',*,*,#21322,.F.);
#31058=ORIENTED_EDGE('',*,*,#21324,.F.);
#31059=ORIENTED_EDGE('',*,*,#21324,.T.);
#31060=ORIENTED_EDGE('',*,*,#21320,.F.);
#31061=ORIENTED_EDGE('',*,*,#21325,.T.);
#31062=ORIENTED_EDGE('',*,*,#21326,.T.);
#31063=ORIENTED_EDGE('',*,*,#21327,.T.);
#31064=ORIENTED_EDGE('',*,*,#21328,.F.);
#31065=ORIENTED_EDGE('',*,*,#21329,.T.);
#31066=ORIENTED_EDGE('',*,*,#21330,.F.);
#31067=ORIENTED_EDGE('',*,*,#21331,.T.);
#31068=ORIENTED_EDGE('',*,*,#21332,.F.);
#31069=ORIENTED_EDGE('',*,*,#21230,.T.);
#31070=ORIENTED_EDGE('',*,*,#21233,.F.);
#31071=ORIENTED_EDGE('',*,*,#21226,.T.);
#31072=ORIENTED_EDGE('',*,*,#21204,.T.);
#31073=ORIENTED_EDGE('',*,*,#21201,.T.);
#31074=ORIENTED_EDGE('',*,*,#21198,.T.);
#31075=ORIENTED_EDGE('',*,*,#21219,.T.);
#31076=ORIENTED_EDGE('',*,*,#21223,.F.);
#31077=ORIENTED_EDGE('',*,*,#21333,.T.);
#31078=ORIENTED_EDGE('',*,*,#21243,.T.);
#31079=ORIENTED_EDGE('',*,*,#21334,.F.);
#31080=ORIENTED_EDGE('',*,*,#21335,.F.);
#31081=ORIENTED_EDGE('',*,*,#21334,.T.);
#31082=ORIENTED_EDGE('',*,*,#21250,.T.);
#31083=ORIENTED_EDGE('',*,*,#21336,.F.);
#31084=ORIENTED_EDGE('',*,*,#21337,.F.);
#31085=ORIENTED_EDGE('',*,*,#21336,.T.);
#31086=ORIENTED_EDGE('',*,*,#21253,.T.);
#31087=ORIENTED_EDGE('',*,*,#21338,.F.);
#31088=ORIENTED_EDGE('',*,*,#21339,.F.);
#31089=ORIENTED_EDGE('',*,*,#21338,.T.);
#31090=ORIENTED_EDGE('',*,*,#21258,.T.);
#31091=ORIENTED_EDGE('',*,*,#21340,.F.);
#31092=ORIENTED_EDGE('',*,*,#21341,.F.);
#31093=ORIENTED_EDGE('',*,*,#21340,.T.);
#31094=ORIENTED_EDGE('',*,*,#21261,.T.);
#31095=ORIENTED_EDGE('',*,*,#21342,.F.);
#31096=ORIENTED_EDGE('',*,*,#21343,.F.);
#31097=ORIENTED_EDGE('',*,*,#21344,.T.);
#31098=ORIENTED_EDGE('',*,*,#21270,.T.);
#31099=ORIENTED_EDGE('',*,*,#21345,.F.);
#31100=ORIENTED_EDGE('',*,*,#21346,.F.);
#31101=ORIENTED_EDGE('',*,*,#21345,.T.);
#31102=ORIENTED_EDGE('',*,*,#21275,.T.);
#31103=ORIENTED_EDGE('',*,*,#21193,.F.);
#31104=ORIENTED_EDGE('',*,*,#21347,.F.);
#31105=ORIENTED_EDGE('',*,*,#21195,.T.);
#31106=ORIENTED_EDGE('',*,*,#21285,.T.);
#31107=ORIENTED_EDGE('',*,*,#21348,.F.);
#31108=ORIENTED_EDGE('',*,*,#21349,.F.);
#31109=ORIENTED_EDGE('',*,*,#21348,.T.);
#31110=ORIENTED_EDGE('',*,*,#21288,.T.);
#31111=ORIENTED_EDGE('',*,*,#21350,.F.);
#31112=ORIENTED_EDGE('',*,*,#21351,.F.);
#31113=ORIENTED_EDGE('',*,*,#21352,.T.);
#31114=ORIENTED_EDGE('',*,*,#21353,.T.);
#31115=ORIENTED_EDGE('',*,*,#21354,.F.);
#31116=ORIENTED_EDGE('',*,*,#21289,.F.);
#31117=ORIENTED_EDGE('',*,*,#21355,.T.);
#31118=ORIENTED_EDGE('',*,*,#21356,.T.);
#31119=ORIENTED_EDGE('',*,*,#21352,.F.);
#31120=ORIENTED_EDGE('',*,*,#21303,.F.);
#31121=ORIENTED_EDGE('',*,*,#21357,.T.);
#31122=ORIENTED_EDGE('',*,*,#21358,.T.);
#31123=ORIENTED_EDGE('',*,*,#21355,.F.);
#31124=ORIENTED_EDGE('',*,*,#21310,.F.);
#31125=ORIENTED_EDGE('',*,*,#21359,.T.);
#31126=ORIENTED_EDGE('',*,*,#21360,.T.);
#31127=ORIENTED_EDGE('',*,*,#21357,.F.);
#31128=ORIENTED_EDGE('',*,*,#21314,.F.);
#31129=ORIENTED_EDGE('',*,*,#21361,.T.);
#31130=ORIENTED_EDGE('',*,*,#21362,.T.);
#31131=ORIENTED_EDGE('',*,*,#21359,.F.);
#31132=ORIENTED_EDGE('',*,*,#21318,.F.);
#31133=ORIENTED_EDGE('',*,*,#21363,.T.);
#31134=ORIENTED_EDGE('',*,*,#21364,.T.);
#31135=ORIENTED_EDGE('',*,*,#21361,.F.);
#31136=ORIENTED_EDGE('',*,*,#21323,.F.);
#31137=ORIENTED_EDGE('',*,*,#21365,.T.);
#31138=ORIENTED_EDGE('',*,*,#21366,.T.);
#31139=ORIENTED_EDGE('',*,*,#21363,.F.);
#31140=ORIENTED_EDGE('',*,*,#21326,.F.);
#31141=ORIENTED_EDGE('',*,*,#21346,.T.);
#31142=ORIENTED_EDGE('',*,*,#21347,.T.);
#31143=ORIENTED_EDGE('',*,*,#21192,.T.);
#31144=ORIENTED_EDGE('',*,*,#21349,.T.);
#31145=ORIENTED_EDGE('',*,*,#21351,.T.);
#31146=ORIENTED_EDGE('',*,*,#21367,.F.);
#31147=ORIENTED_EDGE('',*,*,#21353,.F.);
#31148=ORIENTED_EDGE('',*,*,#21356,.F.);
#31149=ORIENTED_EDGE('',*,*,#21358,.F.);
#31150=ORIENTED_EDGE('',*,*,#21360,.F.);
#31151=ORIENTED_EDGE('',*,*,#21362,.F.);
#31152=ORIENTED_EDGE('',*,*,#21364,.F.);
#31153=ORIENTED_EDGE('',*,*,#21366,.F.);
#31154=ORIENTED_EDGE('',*,*,#21368,.F.);
#31155=ORIENTED_EDGE('',*,*,#21335,.T.);
#31156=ORIENTED_EDGE('',*,*,#21337,.T.);
#31157=ORIENTED_EDGE('',*,*,#21339,.T.);
#31158=ORIENTED_EDGE('',*,*,#21341,.T.);
#31159=ORIENTED_EDGE('',*,*,#21343,.T.);
#31160=ORIENTED_EDGE('',*,*,#21369,.F.);
#31161=ORIENTED_EDGE('',*,*,#21350,.T.);
#31162=ORIENTED_EDGE('',*,*,#21370,.F.);
#31163=ORIENTED_EDGE('',*,*,#21371,.F.);
#31164=ORIENTED_EDGE('',*,*,#21372,.F.);
#31165=ORIENTED_EDGE('',*,*,#21372,.T.);
#31166=ORIENTED_EDGE('',*,*,#21354,.T.);
#31167=ORIENTED_EDGE('',*,*,#21373,.T.);
#31168=ORIENTED_EDGE('',*,*,#21374,.F.);
#31169=ORIENTED_EDGE('',*,*,#21375,.F.);
#31170=ORIENTED_EDGE('',*,*,#21375,.T.);
#31171=ORIENTED_EDGE('',*,*,#21376,.F.);
#31172=ORIENTED_EDGE('',*,*,#21377,.F.);
#31173=ORIENTED_EDGE('',*,*,#21373,.F.);
#31174=ORIENTED_EDGE('',*,*,#21367,.T.);
#31175=ORIENTED_EDGE('',*,*,#21371,.T.);
#31176=ORIENTED_EDGE('',*,*,#21378,.T.);
#31177=ORIENTED_EDGE('',*,*,#21281,.T.);
#31178=ORIENTED_EDGE('',*,*,#21379,.F.);
#31179=ORIENTED_EDGE('',*,*,#21380,.F.);
#31180=ORIENTED_EDGE('',*,*,#21370,.T.);
#31181=ORIENTED_EDGE('',*,*,#21287,.T.);
#31182=ORIENTED_EDGE('',*,*,#21378,.F.);
#31183=ORIENTED_EDGE('',*,*,#21381,.F.);
#31184=ORIENTED_EDGE('',*,*,#21376,.T.);
#31185=ORIENTED_EDGE('',*,*,#21374,.T.);
#31186=ORIENTED_EDGE('',*,*,#21382,.T.);
#31187=ORIENTED_EDGE('',*,*,#21383,.F.);
#31188=ORIENTED_EDGE('',*,*,#21290,.F.);
#31189=ORIENTED_EDGE('',*,*,#21383,.T.);
#31190=ORIENTED_EDGE('',*,*,#21384,.T.);
#31191=ORIENTED_EDGE('',*,*,#21385,.F.);
#31192=ORIENTED_EDGE('',*,*,#21293,.F.);
#31193=ORIENTED_EDGE('',*,*,#21385,.T.);
#31194=ORIENTED_EDGE('',*,*,#21386,.T.);
#31195=ORIENTED_EDGE('',*,*,#21387,.F.);
#31196=ORIENTED_EDGE('',*,*,#21300,.F.);
#31197=ORIENTED_EDGE('',*,*,#21388,.T.);
#31198=ORIENTED_EDGE('',*,*,#21331,.F.);
#31199=ORIENTED_EDGE('',*,*,#21389,.F.);
#31200=ORIENTED_EDGE('',*,*,#21386,.F.);
#31201=ORIENTED_EDGE('',*,*,#21384,.F.);
#31202=ORIENTED_EDGE('',*,*,#21382,.F.);
#31203=ORIENTED_EDGE('',*,*,#21377,.T.);
#31204=ORIENTED_EDGE('',*,*,#21381,.T.);
#31205=ORIENTED_EDGE('',*,*,#21380,.T.);
#31206=ORIENTED_EDGE('',*,*,#21387,.T.);
#31207=ORIENTED_EDGE('',*,*,#21390,.T.);
#31208=ORIENTED_EDGE('',*,*,#21391,.F.);
#31209=ORIENTED_EDGE('',*,*,#21301,.F.);
#31210=ORIENTED_EDGE('',*,*,#21389,.T.);
#31211=ORIENTED_EDGE('',*,*,#21330,.T.);
#31212=ORIENTED_EDGE('',*,*,#21392,.F.);
#31213=ORIENTED_EDGE('',*,*,#21390,.F.);
#31214=ORIENTED_EDGE('',*,*,#21393,.T.);
#31215=ORIENTED_EDGE('',*,*,#21394,.F.);
#31216=ORIENTED_EDGE('',*,*,#21394,.T.);
#31217=ORIENTED_EDGE('',*,*,#21395,.T.);
#31218=ORIENTED_EDGE('',*,*,#21333,.F.);
#31219=ORIENTED_EDGE('',*,*,#21396,.F.);
#31220=ORIENTED_EDGE('',*,*,#21397,.T.);
#31221=ORIENTED_EDGE('',*,*,#21398,.T.);
#31222=ORIENTED_EDGE('',*,*,#21399,.F.);
#31223=ORIENTED_EDGE('',*,*,#21399,.T.);
#31224=ORIENTED_EDGE('',*,*,#21365,.F.);
#31225=ORIENTED_EDGE('',*,*,#21400,.F.);
#31226=ORIENTED_EDGE('',*,*,#21396,.T.);
#31227=ORIENTED_EDGE('',*,*,#21368,.T.);
#31228=ORIENTED_EDGE('',*,*,#21398,.F.);
#31229=ORIENTED_EDGE('',*,*,#21401,.T.);
#31230=ORIENTED_EDGE('',*,*,#21239,.T.);
#31231=ORIENTED_EDGE('',*,*,#21402,.F.);
#31232=ORIENTED_EDGE('',*,*,#21403,.F.);
#31233=ORIENTED_EDGE('',*,*,#21402,.T.);
#31234=ORIENTED_EDGE('',*,*,#21244,.T.);
#31235=ORIENTED_EDGE('',*,*,#21395,.F.);
#31236=ORIENTED_EDGE('',*,*,#21393,.F.);
#31237=ORIENTED_EDGE('',*,*,#21404,.F.);
#31238=ORIENTED_EDGE('',*,*,#21391,.T.);
#31239=ORIENTED_EDGE('',*,*,#21405,.T.);
#31240=ORIENTED_EDGE('',*,*,#21406,.F.);
#31241=ORIENTED_EDGE('',*,*,#21302,.F.);
#31242=ORIENTED_EDGE('',*,*,#21406,.T.);
#31243=ORIENTED_EDGE('',*,*,#21407,.T.);
#31244=ORIENTED_EDGE('',*,*,#21408,.F.);
#31245=ORIENTED_EDGE('',*,*,#21319,.F.);
#31246=ORIENTED_EDGE('',*,*,#21408,.T.);
#31247=ORIENTED_EDGE('',*,*,#21409,.T.);
#31248=ORIENTED_EDGE('',*,*,#21397,.F.);
#31249=ORIENTED_EDGE('',*,*,#21325,.F.);
#31250=ORIENTED_EDGE('',*,*,#21392,.T.);
#31251=ORIENTED_EDGE('',*,*,#21329,.F.);
#31252=ORIENTED_EDGE('',*,*,#21410,.F.);
#31253=ORIENTED_EDGE('',*,*,#21403,.T.);
#31254=ORIENTED_EDGE('',*,*,#21404,.T.);
#31255=ORIENTED_EDGE('',*,*,#21400,.T.);
#31256=ORIENTED_EDGE('',*,*,#21409,.F.);
#31257=ORIENTED_EDGE('',*,*,#21407,.F.);
#31258=ORIENTED_EDGE('',*,*,#21405,.F.);
#31259=ORIENTED_EDGE('',*,*,#21411,.T.);
#31260=ORIENTED_EDGE('',*,*,#21266,.T.);
#31261=ORIENTED_EDGE('',*,*,#21412,.F.);
#31262=ORIENTED_EDGE('',*,*,#21413,.F.);
#31263=ORIENTED_EDGE('',*,*,#21379,.T.);
#31264=ORIENTED_EDGE('',*,*,#21280,.T.);
#31265=ORIENTED_EDGE('',*,*,#21411,.F.);
#31266=ORIENTED_EDGE('',*,*,#21414,.F.);
#31267=ORIENTED_EDGE('',*,*,#21415,.T.);
#31268=ORIENTED_EDGE('',*,*,#21332,.T.);
#31269=ORIENTED_EDGE('',*,*,#21388,.F.);
#31270=ORIENTED_EDGE('',*,*,#21414,.T.);
#31271=ORIENTED_EDGE('',*,*,#21413,.T.);
#31272=ORIENTED_EDGE('',*,*,#21416,.T.);
#31273=ORIENTED_EDGE('',*,*,#21237,.T.);
#31274=ORIENTED_EDGE('',*,*,#21417,.F.);
#31275=ORIENTED_EDGE('',*,*,#21418,.F.);
#31276=ORIENTED_EDGE('',*,*,#21417,.T.);
#31277=ORIENTED_EDGE('',*,*,#21240,.T.);
#31278=ORIENTED_EDGE('',*,*,#21401,.F.);
#31279=ORIENTED_EDGE('',*,*,#21419,.F.);
#31280=ORIENTED_EDGE('',*,*,#21410,.T.);
#31281=ORIENTED_EDGE('',*,*,#21328,.T.);
#31282=ORIENTED_EDGE('',*,*,#21420,.F.);
#31283=ORIENTED_EDGE('',*,*,#21418,.T.);
#31284=ORIENTED_EDGE('',*,*,#21419,.T.);
#31285=ORIENTED_EDGE('',*,*,#21342,.T.);
#31286=ORIENTED_EDGE('',*,*,#21421,.F.);
#31287=ORIENTED_EDGE('',*,*,#21422,.F.);
#31288=ORIENTED_EDGE('',*,*,#21423,.F.);
#31289=ORIENTED_EDGE('',*,*,#21423,.T.);
#31290=ORIENTED_EDGE('',*,*,#21424,.T.);
#31291=ORIENTED_EDGE('',*,*,#21425,.F.);
#31292=ORIENTED_EDGE('',*,*,#21425,.T.);
#31293=ORIENTED_EDGE('',*,*,#21426,.T.);
#31294=ORIENTED_EDGE('',*,*,#21344,.F.);
#31295=ORIENTED_EDGE('',*,*,#21427,.F.);
#31296=ORIENTED_EDGE('',*,*,#21369,.T.);
#31297=ORIENTED_EDGE('',*,*,#21422,.T.);
#31298=ORIENTED_EDGE('',*,*,#21428,.F.);
#31299=ORIENTED_EDGE('',*,*,#21427,.T.);
#31300=ORIENTED_EDGE('',*,*,#21429,.T.);
#31301=ORIENTED_EDGE('',*,*,#21238,.T.);
#31302=ORIENTED_EDGE('',*,*,#21416,.F.);
#31303=ORIENTED_EDGE('',*,*,#21430,.F.);
#31304=ORIENTED_EDGE('',*,*,#21431,.T.);
#31305=ORIENTED_EDGE('',*,*,#21254,.T.);
#31306=ORIENTED_EDGE('',*,*,#21429,.F.);
#31307=ORIENTED_EDGE('',*,*,#21432,.F.);
#31308=ORIENTED_EDGE('',*,*,#21421,.T.);
#31309=ORIENTED_EDGE('',*,*,#21260,.T.);
#31310=ORIENTED_EDGE('',*,*,#21431,.F.);
#31311=ORIENTED_EDGE('',*,*,#21433,.F.);
#31312=ORIENTED_EDGE('',*,*,#21412,.T.);
#31313=ORIENTED_EDGE('',*,*,#21265,.T.);
#31314=ORIENTED_EDGE('',*,*,#21434,.F.);
#31315=ORIENTED_EDGE('',*,*,#21435,.F.);
#31316=ORIENTED_EDGE('',*,*,#21434,.T.);
#31317=ORIENTED_EDGE('',*,*,#21267,.T.);
#31318=ORIENTED_EDGE('',*,*,#21436,.F.);
#31319=ORIENTED_EDGE('',*,*,#21437,.F.);
#31320=ORIENTED_EDGE('',*,*,#21436,.T.);
#31321=ORIENTED_EDGE('',*,*,#21271,.T.);
#31322=ORIENTED_EDGE('',*,*,#21426,.F.);
#31323=ORIENTED_EDGE('',*,*,#21424,.F.);
#31324=ORIENTED_EDGE('',*,*,#21438,.F.);
#31325=ORIENTED_EDGE('',*,*,#21428,.T.);
#31326=ORIENTED_EDGE('',*,*,#21433,.T.);
#31327=ORIENTED_EDGE('',*,*,#21432,.T.);
#31328=ORIENTED_EDGE('',*,*,#21430,.T.);
#31329=ORIENTED_EDGE('',*,*,#21420,.T.);
#31330=ORIENTED_EDGE('',*,*,#21327,.F.);
#31331=ORIENTED_EDGE('',*,*,#21415,.F.);
#31332=ORIENTED_EDGE('',*,*,#21435,.T.);
#31333=ORIENTED_EDGE('',*,*,#21437,.T.);
#31334=ORIENTED_EDGE('',*,*,#21438,.T.);
#33933=ADVANCED_FACE('',(#5185),#411,.T.);
#33934=ADVANCED_FACE('',(#5186),#3191,.F.);
#33935=ADVANCED_FACE('',(#5187),#3192,.F.);
#33936=ADVANCED_FACE('',(#5188),#3193,.F.);
#33937=ADVANCED_FACE('',(#5189),#412,.F.);
#33938=ADVANCED_FACE('',(#5190),#1242,.T.);
#33939=ADVANCED_FACE('',(#5191),#413,.F.);
#33940=ADVANCED_FACE('',(#5192),#2440,.T.);
#33941=ADVANCED_FACE('',(#5193),#414,.F.);
#33942=ADVANCED_FACE('',(#5194),#3194,.F.);
#33943=ADVANCED_FACE('',(#5195),#415,.F.);
#33944=ADVANCED_FACE('',(#5196),#3195,.F.);
#33945=ADVANCED_FACE('',(#5197),#416,.F.);
#33946=ADVANCED_FACE('',(#5198),#3196,.F.);
#33947=ADVANCED_FACE('',(#5199),#3197,.F.);
#33948=ADVANCED_FACE('',(#5200),#417,.F.);
#33949=ADVANCED_FACE('',(#5201),#1243,.T.);
#33950=ADVANCED_FACE('',(#5202),#3198,.F.);
#33951=ADVANCED_FACE('',(#5203),#2441,.T.);
#33952=ADVANCED_FACE('',(#5204),#3199,.F.);
#33953=ADVANCED_FACE('',(#5205),#2442,.F.);
#33954=ADVANCED_FACE('',(#5206),#418,.F.);
#33955=ADVANCED_FACE('',(#5207),#847,.F.);
#33956=ADVANCED_FACE('',(#5208),#3200,.F.);
#33957=ADVANCED_FACE('',(#5209),#3201,.T.);
#33958=ADVANCED_FACE('',(#5210),#3202,.F.);
#33959=ADVANCED_FACE('',(#5211),#848,.F.);
#33960=ADVANCED_FACE('',(#5212),#3203,.F.);
#33961=ADVANCED_FACE('',(#5213),#2443,.T.);
#33962=ADVANCED_FACE('',(#5214),#2444,.T.);
#33963=ADVANCED_FACE('',(#5215),#3204,.F.);
#33964=ADVANCED_FACE('',(#5216),#2445,.F.);
#33965=ADVANCED_FACE('',(#5217),#849,.F.);
#33966=ADVANCED_FACE('',(#5218),#3205,.F.);
#33967=ADVANCED_FACE('',(#5219),#3206,.T.);
#33968=ADVANCED_FACE('',(#5220),#419,.F.);
#33969=ADVANCED_FACE('',(#5221),#3207,.F.);
#33970=ADVANCED_FACE('',(#5222),#850,.F.);
#33971=ADVANCED_FACE('',(#5223),#3208,.F.);
#33972=ADVANCED_FACE('',(#5224),#2446,.T.);
#33973=ADVANCED_FACE('',(#5225),#2447,.F.);
#33974=ADVANCED_FACE('',(#5226),#3209,.F.);
#33975=ADVANCED_FACE('',(#5227),#2448,.T.);
#33976=ADVANCED_FACE('',(#5228),#3210,.F.);
#33977=ADVANCED_FACE('',(#5229),#851,.F.);
#33978=ADVANCED_FACE('',(#5230),#420,.F.);
#33979=ADVANCED_FACE('',(#5231),#3211,.T.);
#33980=ADVANCED_FACE('',(#5232),#421,.F.);
#33981=ADVANCED_FACE('',(#5233),#3212,.T.);
#33982=ADVANCED_FACE('',(#5234),#422,.F.);
#33983=ADVANCED_FACE('',(#5235),#3213,.T.);
#33984=ADVANCED_FACE('',(#5236),#3214,.F.);
#33985=ADVANCED_FACE('',(#5237),#852,.F.);
#33986=ADVANCED_FACE('',(#5238),#3215,.F.);
#33987=ADVANCED_FACE('',(#5239),#2449,.T.);
#33988=ADVANCED_FACE('',(#5240,#1315),#2450,.T.);
#33989=ADVANCED_FACE('',(#5241),#3216,.T.);
#33990=ADVANCED_FACE('',(#5242),#423,.T.);
#33991=ADVANCED_FACE('',(#5243),#424,.T.);
#33992=ADVANCED_FACE('',(#5244),#425,.T.);
#33993=ADVANCED_FACE('',(#5245),#3217,.T.);
#33994=ADVANCED_FACE('',(#5246),#3218,.T.);
#33995=ADVANCED_FACE('',(#5247),#426,.T.);
#33996=ADVANCED_FACE('',(#5248),#427,.T.);
#33997=ADVANCED_FACE('',(#5249),#3219,.T.);
#33998=ADVANCED_FACE('',(#5250),#3220,.T.);
#33999=ADVANCED_FACE('',(#5251),#428,.T.);
#34000=ADVANCED_FACE('',(#5252),#429,.T.);
#34001=ADVANCED_FACE('',(#5253),#430,.T.);
#34002=ADVANCED_FACE('',(#5254),#431,.T.);
#34003=ADVANCED_FACE('',(#5255),#432,.T.);
#34004=ADVANCED_FACE('',(#5256),#3221,.T.);
#34005=ADVANCED_FACE('',(#5257),#2451,.F.);
#34006=ADVANCED_FACE('',(#5258),#853,.T.);
#34007=ADVANCED_FACE('',(#5259),#854,.T.);
#34008=ADVANCED_FACE('',(#5260),#433,.T.);
#34009=ADVANCED_FACE('',(#5261),#1244,.T.);
#34010=ADVANCED_FACE('',(#5262),#3222,.T.);
#34011=ADVANCED_FACE('',(#5263),#3223,.T.);
#34012=ADVANCED_FACE('',(#5264),#1245,.T.);
#34013=ADVANCED_FACE('',(#5265),#434,.T.);
#34014=ADVANCED_FACE('',(#5266),#3224,.T.);
#34015=ADVANCED_FACE('',(#5267),#435,.T.);
#34016=ADVANCED_FACE('',(#5268),#3225,.T.);
#34017=ADVANCED_FACE('',(#5269),#855,.T.);
#34018=ADVANCED_FACE('',(#5270),#856,.T.);
#34019=ADVANCED_FACE('',(#5271),#436,.T.);
#34020=ADVANCED_FACE('',(#5272),#1246,.T.);
#34021=ADVANCED_FACE('',(#5273),#3226,.T.);
#34022=ADVANCED_FACE('',(#5274),#437,.T.);
#34023=ADVANCED_FACE('',(#5275),#1247,.T.);
#34024=ADVANCED_FACE('',(#5276),#3227,.T.);
#34025=ADVANCED_FACE('',(#5277),#3228,.T.);
#34026=ADVANCED_FACE('',(#5278),#438,.T.);
#34027=ADVANCED_FACE('',(#5279),#1248,.T.);
#34028=ADVANCED_FACE('',(#5280),#3229,.T.);
#34029=ADVANCED_FACE('',(#5281),#439,.T.);
#34030=ADVANCED_FACE('',(#5282),#1249,.T.);
#34031=ADVANCED_FACE('',(#5283),#3230,.T.);
#34032=ADVANCED_FACE('',(#5284),#857,.T.);
#34033=ADVANCED_FACE('',(#5285),#858,.T.);
#34034=ADVANCED_FACE('',(#5286),#440,.T.);
#34035=ADVANCED_FACE('',(#5287),#441,.T.);
#34036=ADVANCED_FACE('',(#5288),#1250,.T.);
#34037=ADVANCED_FACE('',(#5289),#3231,.T.);
#34038=ADVANCED_FACE('',(#5290),#442,.T.);
#34039=ADVANCED_FACE('',(#5291),#1251,.T.);
#34040=ADVANCED_FACE('',(#5292),#3232,.T.);
#34041=ADVANCED_FACE('',(#5293),#3233,.T.);
#34177=CLOSED_SHELL('',(#33933,#33934,#33935,#33936,#33937,#33938,#33939,
#33940,#33941,#33942,#33943,#33944,#33945,#33946,#33947,#33948,#33949,#33950,
#33951,#33952,#33953,#33954,#33955,#33956,#33957,#33958,#33959,#33960,#33961,
#33962,#33963,#33964,#33965,#33966,#33967,#33968,#33969,#33970,#33971,#33972,
#33973,#33974,#33975,#33976,#33977,#33978,#33979,#33980,#33981,#33982,#33983,
#33984,#33985,#33986,#33987,#33988,#33989,#33990,#33991,#33992,#33993,#33994,
#33995,#33996,#33997,#33998,#33999,#34000,#34001,#34002,#34003,#34004,#34005,
#34006,#34007,#34008,#34009,#34010,#34011,#34012,#34013,#34014,#34015,#34016,
#34017,#34018,#34019,#34020,#34021,#34022,#34023,#34024,#34025,#34026,#34027,
#34028,#34029,#34030,#34031,#34032,#34033,#34034,#34035,#34036,#34037,#34038,
#34039,#34040,#34041));
#38088=AXIS2_PLACEMENT_3D('',#95794,#47795,#47796);
#38089=AXIS2_PLACEMENT_3D('',#95795,#47797,#47798);
#38090=AXIS2_PLACEMENT_3D('',#95798,#47799,#47800);
#38091=AXIS2_PLACEMENT_3D('',#95800,#47801,#47802);
#38092=AXIS2_PLACEMENT_3D('',#95802,#47803,#47804);
#38093=AXIS2_PLACEMENT_3D('',#95803,#47805,#47806);
#38094=AXIS2_PLACEMENT_3D('',#95804,#47807,#47808);
#38095=AXIS2_PLACEMENT_3D('',#95807,#47809,#47810);
#38096=AXIS2_PLACEMENT_3D('',#95811,#47812,#47813);
#38097=AXIS2_PLACEMENT_3D('',#95813,#47815,#47816);
#38098=AXIS2_PLACEMENT_3D('',#95815,#47817,#47818);
#38099=AXIS2_PLACEMENT_3D('',#95817,#47819,#47820);
#38100=AXIS2_PLACEMENT_3D('',#95819,#47822,#47823);
#38101=AXIS2_PLACEMENT_3D('',#95821,#47824,#47825);
#38102=AXIS2_PLACEMENT_3D('',#95823,#47826,#47827);
#38103=AXIS2_PLACEMENT_3D('',#95825,#47829,#47830);
#38104=AXIS2_PLACEMENT_3D('',#95883,#47831,#47832);
#38105=AXIS2_PLACEMENT_3D('',#95884,#47833,#47834);
#38106=AXIS2_PLACEMENT_3D('',#95946,#47835,#47836);
#38107=AXIS2_PLACEMENT_3D('',#95948,#47837,#47838);
#38108=AXIS2_PLACEMENT_3D('',#95949,#47839,#47840);
#38109=AXIS2_PLACEMENT_3D('',#95950,#47841,#47842);
#38110=AXIS2_PLACEMENT_3D('',#95953,#47843,#47844);
#38111=AXIS2_PLACEMENT_3D('',#95954,#47845,#47846);
#38112=AXIS2_PLACEMENT_3D('',#95956,#47847,#47848);
#38113=AXIS2_PLACEMENT_3D('',#95957,#47849,#47850);
#38114=AXIS2_PLACEMENT_3D('',#95958,#47851,#47852);
#38115=AXIS2_PLACEMENT_3D('',#95960,#47853,#47854);
#38116=AXIS2_PLACEMENT_3D('',#95961,#47855,#47856);
#38117=AXIS2_PLACEMENT_3D('',#95962,#47857,#47858);
#38118=AXIS2_PLACEMENT_3D('',#95965,#47860,#47861);
#38119=AXIS2_PLACEMENT_3D('',#95966,#47862,#47863);
#38120=AXIS2_PLACEMENT_3D('',#95973,#47864,#47865);
#38121=AXIS2_PLACEMENT_3D('',#95974,#47866,#47867);
#38122=AXIS2_PLACEMENT_3D('',#95977,#47869,#47870);
#38123=AXIS2_PLACEMENT_3D('',#95978,#47871,#47872);
#38124=AXIS2_PLACEMENT_3D('',#95980,#47873,#47874);
#38125=AXIS2_PLACEMENT_3D('',#95981,#47875,#47876);
#38126=AXIS2_PLACEMENT_3D('',#95982,#47877,#47878);
#38127=AXIS2_PLACEMENT_3D('',#95984,#47879,#47880);
#38128=AXIS2_PLACEMENT_3D('',#95986,#47882,#47883);
#38129=AXIS2_PLACEMENT_3D('',#95988,#47884,#47885);
#38130=AXIS2_PLACEMENT_3D('',#95991,#47887,#47888);
#38131=AXIS2_PLACEMENT_3D('',#95992,#47889,#47890);
#38132=AXIS2_PLACEMENT_3D('',#96048,#47891,#47892);
#38133=AXIS2_PLACEMENT_3D('',#96079,#47893,#47894);
#38134=AXIS2_PLACEMENT_3D('',#96080,#47895,#47896);
#38135=AXIS2_PLACEMENT_3D('',#96081,#47897,#47898);
#38136=AXIS2_PLACEMENT_3D('',#96086,#47900,#47901);
#38137=AXIS2_PLACEMENT_3D('',#96090,#47903,#47904);
#38138=AXIS2_PLACEMENT_3D('',#96091,#47905,#47906);
#38139=AXIS2_PLACEMENT_3D('',#96092,#47907,#47908);
#38140=AXIS2_PLACEMENT_3D('',#96124,#47909,#47910);
#38141=AXIS2_PLACEMENT_3D('',#96126,#47912,#47913);
#38142=AXIS2_PLACEMENT_3D('',#96132,#47917,#47918);
#38143=AXIS2_PLACEMENT_3D('',#96134,#47919,#47920);
#38144=AXIS2_PLACEMENT_3D('',#96136,#47921,#47922);
#38145=AXIS2_PLACEMENT_3D('',#96137,#47923,#47924);
#38146=AXIS2_PLACEMENT_3D('',#96138,#47925,#47926);
#38147=AXIS2_PLACEMENT_3D('',#96139,#47927,#47928);
#38148=AXIS2_PLACEMENT_3D('',#96140,#47929,#47930);
#38149=AXIS2_PLACEMENT_3D('',#96142,#47931,#47932);
#38150=AXIS2_PLACEMENT_3D('',#96144,#47934,#47935);
#38151=AXIS2_PLACEMENT_3D('',#96147,#47937,#47938);
#38152=AXIS2_PLACEMENT_3D('',#96148,#47939,#47940);
#38153=AXIS2_PLACEMENT_3D('',#96189,#47942,#47943);
#38154=AXIS2_PLACEMENT_3D('',#96190,#47944,#47945);
#38155=AXIS2_PLACEMENT_3D('',#96191,#47946,#47947);
#38156=AXIS2_PLACEMENT_3D('',#96192,#47948,#47949);
#38157=AXIS2_PLACEMENT_3D('',#96194,#47950,#47951);
#38158=AXIS2_PLACEMENT_3D('',#96196,#47953,#47954);
#38159=AXIS2_PLACEMENT_3D('',#96200,#47957,#47958);
#38160=AXIS2_PLACEMENT_3D('',#96205,#47960,#47961);
#38161=AXIS2_PLACEMENT_3D('',#96209,#47963,#47964);
#38162=AXIS2_PLACEMENT_3D('',#96210,#47965,#47966);
#38163=AXIS2_PLACEMENT_3D('',#96211,#47967,#47968);
#38164=AXIS2_PLACEMENT_3D('',#96223,#47969,#47970);
#38165=AXIS2_PLACEMENT_3D('',#96225,#47972,#47973);
#38166=AXIS2_PLACEMENT_3D('',#96231,#47977,#47978);
#38167=AXIS2_PLACEMENT_3D('',#96233,#47979,#47980);
#38168=AXIS2_PLACEMENT_3D('',#96234,#47981,#47982);
#38169=AXIS2_PLACEMENT_3D('',#96235,#47983,#47984);
#38170=AXIS2_PLACEMENT_3D('',#96236,#47985,#47986);
#38171=AXIS2_PLACEMENT_3D('',#96238,#47988,#47989);
#38172=AXIS2_PLACEMENT_3D('',#96240,#47990,#47991);
#38173=AXIS2_PLACEMENT_3D('',#96242,#47993,#47994);
#38174=AXIS2_PLACEMENT_3D('',#96243,#47995,#47996);
#38175=AXIS2_PLACEMENT_3D('',#96244,#47997,#47998);
#38176=AXIS2_PLACEMENT_3D('',#96274,#48000,#48001);
#38177=AXIS2_PLACEMENT_3D('',#96275,#48002,#48003);
#38178=AXIS2_PLACEMENT_3D('',#96276,#48004,#48005);
#38179=AXIS2_PLACEMENT_3D('',#96277,#48006,#48007);
#38180=AXIS2_PLACEMENT_3D('',#96279,#48008,#48009);
#38181=AXIS2_PLACEMENT_3D('',#96281,#48011,#48012);
#38182=AXIS2_PLACEMENT_3D('',#96285,#48015,#48016);
#38183=AXIS2_PLACEMENT_3D('',#96294,#48021,#48022);
#38184=AXIS2_PLACEMENT_3D('',#96332,#48024,#48025);
#38185=AXIS2_PLACEMENT_3D('',#96333,#48026,#48027);
#38186=AXIS2_PLACEMENT_3D('',#96338,#48029,#48030);
#38187=AXIS2_PLACEMENT_3D('',#96340,#48031,#48032);
#38188=AXIS2_PLACEMENT_3D('',#96341,#48033,#48034);
#38189=AXIS2_PLACEMENT_3D('',#96343,#48035,#48036);
#38190=AXIS2_PLACEMENT_3D('',#96345,#48037,#48038);
#38191=AXIS2_PLACEMENT_3D('',#96346,#48039,#48040);
#38192=AXIS2_PLACEMENT_3D('',#96347,#48041,#48042);
#38193=AXIS2_PLACEMENT_3D('',#96349,#48043,#48044);
#38194=AXIS2_PLACEMENT_3D('',#96351,#48045,#48046);
#38195=AXIS2_PLACEMENT_3D('',#96353,#48048,#48049);
#38196=AXIS2_PLACEMENT_3D('',#96354,#48050,#48051);
#38197=AXIS2_PLACEMENT_3D('',#96355,#48052,#48053);
#38198=AXIS2_PLACEMENT_3D('',#96357,#48054,#48055);
#38199=AXIS2_PLACEMENT_3D('',#96358,#48056,#48057);
#38200=AXIS2_PLACEMENT_3D('',#96359,#48058,#48059);
#38201=AXIS2_PLACEMENT_3D('',#96362,#48061,#48062);
#38202=AXIS2_PLACEMENT_3D('',#96363,#48063,#48064);
#38203=AXIS2_PLACEMENT_3D('',#96365,#48065,#48066);
#38204=AXIS2_PLACEMENT_3D('',#96366,#48067,#48068);
#38205=AXIS2_PLACEMENT_3D('',#96367,#48069,#48070);
#38206=AXIS2_PLACEMENT_3D('',#96370,#48072,#48073);
#38207=AXIS2_PLACEMENT_3D('',#96371,#48074,#48075);
#38208=AXIS2_PLACEMENT_3D('',#96373,#48076,#48077);
#38209=AXIS2_PLACEMENT_3D('',#96374,#48078,#48079);
#38210=AXIS2_PLACEMENT_3D('',#96375,#48080,#48081);
#38211=AXIS2_PLACEMENT_3D('',#96378,#48083,#48084);
#38212=AXIS2_PLACEMENT_3D('',#96379,#48085,#48086);
#38213=AXIS2_PLACEMENT_3D('',#96404,#48088,#48089);
#38214=AXIS2_PLACEMENT_3D('',#96405,#48090,#48091);
#38215=AXIS2_PLACEMENT_3D('',#96406,#48092,#48093);
#38216=AXIS2_PLACEMENT_3D('',#96407,#48094,#48095);
#38217=AXIS2_PLACEMENT_3D('',#96409,#48096,#48097);
#38218=AXIS2_PLACEMENT_3D('',#96411,#48099,#48100);
#38219=AXIS2_PLACEMENT_3D('',#96415,#48103,#48104);
#38220=AXIS2_PLACEMENT_3D('',#96418,#48105,#48106);
#38221=AXIS2_PLACEMENT_3D('',#96420,#48107,#48108);
#38222=AXIS2_PLACEMENT_3D('',#96422,#48109,#48110);
#38223=AXIS2_PLACEMENT_3D('',#96424,#48111,#48112);
#38224=AXIS2_PLACEMENT_3D('',#96426,#48113,#48114);
#38225=AXIS2_PLACEMENT_3D('',#96427,#48115,#48116);
#38226=AXIS2_PLACEMENT_3D('',#96428,#48117,#48118);
#38227=AXIS2_PLACEMENT_3D('',#96430,#48119,#48120);
#38228=AXIS2_PLACEMENT_3D('',#96432,#48121,#48122);
#38229=AXIS2_PLACEMENT_3D('',#96434,#48124,#48125);
#38230=AXIS2_PLACEMENT_3D('',#96436,#48126,#48127);
#38231=AXIS2_PLACEMENT_3D('',#96437,#48128,#48129);
#38232=AXIS2_PLACEMENT_3D('',#96438,#48130,#48131);
#38233=AXIS2_PLACEMENT_3D('',#96440,#48132,#48133);
#38234=AXIS2_PLACEMENT_3D('',#96441,#48134,#48135);
#38235=AXIS2_PLACEMENT_3D('',#96442,#48136,#48137);
#38236=AXIS2_PLACEMENT_3D('',#96444,#48138,#48139);
#38237=AXIS2_PLACEMENT_3D('',#96445,#48140,#48141);
#38238=AXIS2_PLACEMENT_3D('',#96446,#48142,#48143);
#38239=AXIS2_PLACEMENT_3D('',#96448,#48144,#48145);
#38240=AXIS2_PLACEMENT_3D('',#96450,#48147,#48148);
#38241=AXIS2_PLACEMENT_3D('',#96452,#48149,#48150);
#38242=AXIS2_PLACEMENT_3D('',#96454,#48151,#48152);
#38243=AXIS2_PLACEMENT_3D('',#96456,#48154,#48155);
#38244=AXIS2_PLACEMENT_3D('',#96457,#48156,#48157);
#38245=AXIS2_PLACEMENT_3D('',#96458,#48158,#48159);
#38246=AXIS2_PLACEMENT_3D('',#96460,#48160,#48161);
#38247=AXIS2_PLACEMENT_3D('',#96461,#48162,#48163);
#38248=AXIS2_PLACEMENT_3D('',#96462,#48164,#48165);
#38249=AXIS2_PLACEMENT_3D('',#96464,#48166,#48167);
#38250=AXIS2_PLACEMENT_3D('',#96466,#48169,#48170);
#38251=AXIS2_PLACEMENT_3D('',#96468,#48171,#48172);
#38252=AXIS2_PLACEMENT_3D('',#96471,#48174,#48175);
#38253=AXIS2_PLACEMENT_3D('',#96472,#48176,#48177);
#38254=AXIS2_PLACEMENT_3D('',#96474,#48178,#48179);
#38255=AXIS2_PLACEMENT_3D('',#96475,#48180,#48181);
#38256=AXIS2_PLACEMENT_3D('',#96476,#48182,#48183);
#38257=AXIS2_PLACEMENT_3D('',#96478,#48184,#48185);
#38258=AXIS2_PLACEMENT_3D('',#96479,#48186,#48187);
#38259=AXIS2_PLACEMENT_3D('',#96480,#48188,#48189);
#38260=AXIS2_PLACEMENT_3D('',#96482,#48190,#48191);
#38261=AXIS2_PLACEMENT_3D('',#96483,#48192,#48193);
#38262=AXIS2_PLACEMENT_3D('',#96484,#48194,#48195);
#38263=AXIS2_PLACEMENT_3D('',#96486,#48196,#48197);
#38264=AXIS2_PLACEMENT_3D('',#96487,#48198,#48199);
#38265=AXIS2_PLACEMENT_3D('',#96488,#48200,#48201);
#38266=AXIS2_PLACEMENT_3D('',#96490,#48202,#48203);
#38267=AXIS2_PLACEMENT_3D('',#96491,#48204,#48205);
#38268=AXIS2_PLACEMENT_3D('',#96492,#48206,#48207);
#38269=AXIS2_PLACEMENT_3D('',#96494,#48208,#48209);
#38270=AXIS2_PLACEMENT_3D('',#96496,#48211,#48212);
#38271=AXIS2_PLACEMENT_3D('',#96497,#48213,#48214);
#38272=AXIS2_PLACEMENT_3D('',#96498,#48215,#48216);
#38273=AXIS2_PLACEMENT_3D('',#96499,#48217,#48218);
#38274=AXIS2_PLACEMENT_3D('',#96500,#48219,#48220);
#38275=AXIS2_PLACEMENT_3D('',#96502,#48221,#48222);
#38276=AXIS2_PLACEMENT_3D('',#96503,#48223,#48224);
#38277=AXIS2_PLACEMENT_3D('',#96505,#48225,#48226);
#38278=AXIS2_PLACEMENT_3D('',#96506,#48227,#48228);
#38279=AXIS2_PLACEMENT_3D('',#96508,#48229,#48230);
#38280=AXIS2_PLACEMENT_3D('',#96510,#48231,#48232);
#38281=AXIS2_PLACEMENT_3D('',#96512,#48233,#48234);
#38282=AXIS2_PLACEMENT_3D('',#96513,#48235,#48236);
#38283=AXIS2_PLACEMENT_3D('',#96514,#48237,#48238);
#38284=AXIS2_PLACEMENT_3D('',#96515,#48239,#48240);
#38285=AXIS2_PLACEMENT_3D('',#96598,#48241,#48242);
#38286=AXIS2_PLACEMENT_3D('',#96600,#48243,#48244);
#38287=AXIS2_PLACEMENT_3D('',#96610,#48245,#48246);
#38288=AXIS2_PLACEMENT_3D('',#96612,#48248,#48249);
#38289=AXIS2_PLACEMENT_3D('',#96685,#48251,#48252);
#38290=AXIS2_PLACEMENT_3D('',#96686,#48253,#48254);
#38291=AXIS2_PLACEMENT_3D('',#96688,#48255,#48256);
#38292=AXIS2_PLACEMENT_3D('',#96689,#48257,#48258);
#38293=AXIS2_PLACEMENT_3D('',#96690,#48259,#48260);
#38294=AXIS2_PLACEMENT_3D('',#96693,#48263,#48264);
#38295=AXIS2_PLACEMENT_3D('',#96695,#48265,#48266);
#38296=AXIS2_PLACEMENT_3D('',#96696,#48267,#48268);
#38297=AXIS2_PLACEMENT_3D('',#96697,#48269,#48270);
#38298=AXIS2_PLACEMENT_3D('',#96699,#48272,#48273);
#38299=AXIS2_PLACEMENT_3D('',#96702,#48274,#48275);
#38300=AXIS2_PLACEMENT_3D('',#96704,#48276,#48277);
#38301=AXIS2_PLACEMENT_3D('',#96705,#48278,#48279);
#38302=AXIS2_PLACEMENT_3D('',#96706,#48280,#48281);
#38303=AXIS2_PLACEMENT_3D('',#96707,#48282,#48283);
#38304=AXIS2_PLACEMENT_3D('',#96709,#48284,#48285);
#38305=AXIS2_PLACEMENT_3D('',#96710,#48286,#48287);
#38306=AXIS2_PLACEMENT_3D('',#96712,#48288,#48289);
#38307=AXIS2_PLACEMENT_3D('',#96713,#48290,#48291);
#38308=AXIS2_PLACEMENT_3D('',#96714,#48292,#48293);
#38309=AXIS2_PLACEMENT_3D('',#96797,#48294,#48295);
#38310=AXIS2_PLACEMENT_3D('',#96799,#48296,#48297);
#38311=AXIS2_PLACEMENT_3D('',#96834,#48298,#48299);
#38312=AXIS2_PLACEMENT_3D('',#96836,#48301,#48302);
#38313=AXIS2_PLACEMENT_3D('',#96838,#48303,#48304);
#38314=AXIS2_PLACEMENT_3D('',#96839,#48305,#48306);
#38315=AXIS2_PLACEMENT_3D('',#96941,#48307,#48308);
#38316=AXIS2_PLACEMENT_3D('',#96943,#48310,#48311);
#38317=AXIS2_PLACEMENT_3D('',#96945,#48313,#48314);
#38318=AXIS2_PLACEMENT_3D('',#96947,#48315,#48316);
#38319=AXIS2_PLACEMENT_3D('',#96949,#48317,#48318);
#38320=AXIS2_PLACEMENT_3D('',#96950,#48319,#48320);
#38321=AXIS2_PLACEMENT_3D('',#97000,#48321,#48322);
#38322=AXIS2_PLACEMENT_3D('',#97002,#48324,#48325);
#38323=AXIS2_PLACEMENT_3D('',#97004,#48326,#48327);
#38324=AXIS2_PLACEMENT_3D('',#97006,#48328,#48329);
#38325=AXIS2_PLACEMENT_3D('',#97007,#48330,#48331);
#38326=AXIS2_PLACEMENT_3D('',#97057,#48332,#48333);
#38327=AXIS2_PLACEMENT_3D('',#97059,#48335,#48336);
#38328=AXIS2_PLACEMENT_3D('',#97061,#48337,#48338);
#38329=AXIS2_PLACEMENT_3D('',#97062,#48339,#48340);
#38330=AXIS2_PLACEMENT_3D('',#97064,#48341,#48342);
#38331=AXIS2_PLACEMENT_3D('',#97065,#48343,#48344);
#38332=AXIS2_PLACEMENT_3D('',#97068,#48345,#48346);
#38333=AXIS2_PLACEMENT_3D('',#97070,#48347,#48348);
#38334=AXIS2_PLACEMENT_3D('',#97071,#48349,#48350);
#38335=AXIS2_PLACEMENT_3D('',#97072,#48351,#48352);
#38336=AXIS2_PLACEMENT_3D('',#97073,#48353,#48354);
#38337=AXIS2_PLACEMENT_3D('',#97074,#48355,#48356);
#38338=AXIS2_PLACEMENT_3D('',#97075,#48357,#48358);
#38339=AXIS2_PLACEMENT_3D('',#97077,#48359,#48360);
#38340=AXIS2_PLACEMENT_3D('',#97078,#48361,#48362);
#38341=AXIS2_PLACEMENT_3D('',#97180,#48363,#48364);
#38342=AXIS2_PLACEMENT_3D('',#97182,#48366,#48367);
#38343=AXIS2_PLACEMENT_3D('',#97184,#48368,#48369);
#38344=AXIS2_PLACEMENT_3D('',#97185,#48370,#48371);
#38345=AXIS2_PLACEMENT_3D('',#97327,#48372,#48373);
#38346=AXIS2_PLACEMENT_3D('',#97329,#48375,#48376);
#47795=DIRECTION('axis',(0.,0.,1.));
#47796=DIRECTION('refdir',(1.,0.,0.));
#47797=DIRECTION('center_axis',(-4.22828176385563E-17,-1.,5.82264120529052E-17));
#47798=DIRECTION('ref_axis',(0.809156716779487,0.,0.587592892818354));
#47799=DIRECTION('center_axis',(1.22464679915E-16,1.,3.21507022015E-32));
#47800=DIRECTION('ref_axis',(1.,-1.22464679915E-16,-3.93732545414918E-48));
#47801=DIRECTION('center_axis',(0.814436178114135,-9.97396658637165E-17,
-0.580253144566095));
#47802=DIRECTION('ref_axis',(0.580253144566095,-1.05208313255741E-31,0.814436178114135));
#47803=DIRECTION('center_axis',(1.22464679915E-16,1.,2.46519032882E-32));
#47804=DIRECTION('ref_axis',(1.,-1.22464679915E-16,-3.01898744548495E-48));
#47805=DIRECTION('center_axis',(0.54648608815598,-6.69252438638976E-17,
-0.837468181754969));
#47806=DIRECTION('ref_axis',(0.837468181754969,-2.14539310633749E-32,0.54648608815598));
#47807=DIRECTION('center_axis',(1.22464679914918E-16,1.,2.56032743355287E-29));
#47808=DIRECTION('ref_axis',(0.954110409263768,-1.16844825873972E-16,-0.299455049939928));
#47809=DIRECTION('center_axis',(-1.22464679915E-16,-1.,-3.38963670212E-32));
#47810=DIRECTION('ref_axis',(1.,-1.22464679915E-16,4.23644123317814E-49));
#47811=DIRECTION('',(8.6905911908E-17,1.,0.));
#47812=DIRECTION('center_axis',(1.22464679915E-16,1.,3.21507022015E-32));
#47813=DIRECTION('ref_axis',(1.,-1.22464679915E-16,-3.93732545414918E-48));
#47814=DIRECTION('',(0.,1.,0.));
#47815=DIRECTION('center_axis',(-1.2246467991493E-16,-1.,-2.25761787925393E-29));
#47816=DIRECTION('ref_axis',(0.952002172953202,-1.16586641389025E-16,-0.306091265299064));
#47817=DIRECTION('center_axis',(0.,1.,0.));
#47818=DIRECTION('ref_axis',(0.95200562088917,0.,-0.306080541353786));
#47819=DIRECTION('center_axis',(1.22464679915E-16,1.,3.21507022015E-32));
#47820=DIRECTION('ref_axis',(1.,-1.22464679915E-16,-3.93732545414918E-48));
#47821=DIRECTION('',(2.43336553343E-16,1.,0.));
#47822=DIRECTION('center_axis',(1.22464679915E-16,1.,-1.86877716572514E-30));
#47823=DIRECTION('ref_axis',(0.00535506551034943,-6.5580638364693E-19,0.999985661533894));
#47824=DIRECTION('center_axis',(-1.22464679915E-16,-1.,-2.46519032882E-32));
#47825=DIRECTION('ref_axis',(1.,-1.22464679915E-16,-3.01898744548495E-48));
#47826=DIRECTION('center_axis',(1.22464679915E-16,1.,3.21507022015E-32));
#47827=DIRECTION('ref_axis',(1.,-1.22464679915E-16,-3.93732545414918E-48));
#47828=DIRECTION('',(1.22211438621E-16,1.,0.));
#47829=DIRECTION('center_axis',(-1.59015019497209E-16,-1.,3.16247585529168E-17));
#47830=DIRECTION('ref_axis',(0.756223380296384,-1.38202005618507E-16,-0.654313532714333));
#47831=DIRECTION('center_axis',(-1.22464679915E-16,-1.,-3.21507022015E-32));
#47832=DIRECTION('ref_axis',(1.,-1.22464679915E-16,4.87897920646316E-49));
#47833=DIRECTION('center_axis',(0.654313532714333,-8.01302973477407E-17,
0.756223380296384));
#47834=DIRECTION('ref_axis',(0.756223380296384,1.79722796841309E-32,-0.654313532714333));
#47835=DIRECTION('center_axis',(-1.02993792068947E-16,-1.,4.47814757931693E-17));
#47836=DIRECTION('ref_axis',(0.393698211550324,0.,0.919239750131638));
#47837=DIRECTION('center_axis',(-0.999959189367103,1.22459682054048E-16,
0.00903435666143352));
#47838=DIRECTION('ref_axis',(0.00903435666143352,1.38777878078145E-14,0.999959189367103));
#47839=DIRECTION('center_axis',(-1.22464679915E-16,-1.,-3.21507022015E-32));
#47840=DIRECTION('ref_axis',(1.,-1.22464679915E-16,-3.93732545414918E-48));
#47841=DIRECTION('center_axis',(-1.22464679915E-16,-1.,-3.21507022015E-32));
#47842=DIRECTION('ref_axis',(-1.,1.22464679915E-16,0.));
#47843=DIRECTION('center_axis',(-1.22464679915E-16,-1.,-3.23556230657E-32));
#47844=DIRECTION('ref_axis',(1.,-1.22464679915E-16,4.91007664965853E-49));
#47845=DIRECTION('center_axis',(-1.22464679915E-16,-1.,-2.46519032882E-32));
#47846=DIRECTION('ref_axis',(1.,-1.22464679915E-16,-3.01898744548495E-48));
#47847=DIRECTION('center_axis',(-1.22464679915E-16,-1.,-3.21630300713E-32));
#47848=DIRECTION('ref_axis',(1.,-1.22464679915E-16,-3.93883518277827E-48));
#47849=DIRECTION('center_axis',(-1.22464679915E-16,-1.,-2.46519032882E-32));
#47850=DIRECTION('ref_axis',(1.,-1.22464679915E-16,-3.01898744548495E-48));
#47851=DIRECTION('center_axis',(-5.24303379351633E-17,-1.,6.05964043245936E-17));
#47852=DIRECTION('ref_axis',(-0.756223380296385,0.,-0.654313532714333));
#47853=DIRECTION('center_axis',(-1.22464679915E-16,-1.,-2.46519032882E-32));
#47854=DIRECTION('ref_axis',(1.,-1.22464679915E-16,-3.01898744548495E-48));
#47855=DIRECTION('center_axis',(0.654313532714333,-8.01302973477407E-17,
-0.756223380296384));
#47856=DIRECTION('ref_axis',(0.756223380296384,1.79722796841309E-32,0.654313532714333));
#47857=DIRECTION('center_axis',(-1.22464679914857E-16,-1.,1.23638169675289E-28));
#47858=DIRECTION('ref_axis',(-0.756223380296385,9.2610654212047E-17,-0.654313532714332));
#47859=DIRECTION('',(0.,1.,0.));
#47860=DIRECTION('center_axis',(1.22464679915E-16,1.,3.21507022015E-32));
#47861=DIRECTION('ref_axis',(1.,-1.22464679915E-16,-3.93732545414918E-48));
#47862=DIRECTION('center_axis',(-1.55713156083392E-16,-1.,-2.32366652287783E-17));
#47863=DIRECTION('ref_axis',(-0.871681712672678,1.38202005618507E-16,-0.490072435250165));
#47864=DIRECTION('center_axis',(-1.22464679915E-16,-1.,-3.21507022015E-32));
#47865=DIRECTION('ref_axis',(1.,-1.22464679915E-16,4.01826426994016E-49));
#47866=DIRECTION('center_axis',(-1.22464679914918E-16,-1.,2.55459749524577E-29));
#47867=DIRECTION('ref_axis',(-0.954110409263768,1.16844825873972E-16,-0.299455049939928));
#47868=DIRECTION('',(0.,1.,0.));
#47869=DIRECTION('center_axis',(-1.22464679915E-16,-1.,-3.21507022015E-32));
#47870=DIRECTION('ref_axis',(1.,-1.22464679915E-16,-3.93732545414918E-48));
#47871=DIRECTION('center_axis',(-1.22454684396776E-16,-1.,1.10634444432041E-18));
#47872=DIRECTION('ref_axis',(0.00903435666143093,0.,0.999959189367103));
#47873=DIRECTION('center_axis',(-1.22464679915E-16,-1.,-3.19704370768E-32));
#47874=DIRECTION('ref_axis',(1.,-1.22464679915E-16,-3.91524934335296E-48));
#47875=DIRECTION('center_axis',(-0.999959189367103,1.22459682054048E-16,
-0.00903435666143352));
#47876=DIRECTION('ref_axis',(0.00903435666143352,1.38777878078145E-14,-0.999959189367103));
#47877=DIRECTION('center_axis',(-1.22464679915E-16,-1.,-2.69938341005315E-32));
#47878=DIRECTION('ref_axis',(0.00903435666143093,-1.10638959678011E-18,
0.999959189367103));
#47879=DIRECTION('center_axis',(1.22464679915E-16,1.,3.21507022015E-32));
#47880=DIRECTION('ref_axis',(1.,-1.22464679915E-16,-3.93732545414918E-48));
#47881=DIRECTION('',(1.21668276671E-16,1.,0.));
#47882=DIRECTION('center_axis',(-1.22464679914807E-16,-1.,-1.87465740942333E-28));
#47883=DIRECTION('ref_axis',(-0.717530579084786,8.78721526965739E-17,0.696527004557793));
#47884=DIRECTION('center_axis',(0.,1.,0.));
#47885=DIRECTION('ref_axis',(-0.717538425134005,0.,0.696518921822094));
#47886=DIRECTION('',(0.,1.,0.));
#47887=DIRECTION('center_axis',(1.22464679915E-16,1.,3.21507022015E-32));
#47888=DIRECTION('ref_axis',(1.,-1.22464679915E-16,-3.93732545414918E-48));
#47889=DIRECTION('center_axis',(-1.22454684396776E-16,-1.,-1.10634444432041E-18));
#47890=DIRECTION('ref_axis',(-0.00903435666143093,0.,0.999959189367103));
#47891=DIRECTION('center_axis',(-1.22464679915E-16,-1.,-3.21507022015E-32));
#47892=DIRECTION('ref_axis',(1.,-1.22464679915E-16,-3.93732545414918E-48));
#47893=DIRECTION('center_axis',(-1.22464679915E-16,-1.,-1.86877716572514E-30));
#47894=DIRECTION('ref_axis',(-0.00535506551034943,6.5580638364693E-19,0.999985661533894));
#47895=DIRECTION('center_axis',(-1.22464679915E-16,-1.,-3.21507022015E-32));
#47896=DIRECTION('ref_axis',(1.,-1.22464679915E-16,-3.93732545414918E-48));
#47897=DIRECTION('center_axis',(1.22464679915E-16,1.,3.21507022015E-32));
#47898=DIRECTION('ref_axis',(1.,-1.22464679915E-16,0.));
#47899=DIRECTION('',(-0.734238830876791,0.,0.678891257295807));
#47900=DIRECTION('center_axis',(1.22464679915E-16,1.,2.46519032882E-32));
#47901=DIRECTION('ref_axis',(1.,-1.22464679915E-16,-3.01898744548495E-48));
#47902=DIRECTION('',(0.734238830876791,0.,-0.678891257295807));
#47903=DIRECTION('center_axis',(-1.22464679915E-16,-1.,-3.08148791102E-32));
#47904=DIRECTION('ref_axis',(1.,-1.22464679915E-16,-3.77373430685006E-48));
#47905=DIRECTION('center_axis',(-1.22464679915E-16,-1.,-2.46519032882E-32));
#47906=DIRECTION('ref_axis',(1.,-1.22464679915E-16,2.53931026341659E-48));
#47907=DIRECTION('center_axis',(0.734238830876792,-8.99183234039869E-17,
-0.678891257295808));
#47908=DIRECTION('ref_axis',(-6.60215246505446E-17,-1.,6.10447636296637E-17));
#47909=DIRECTION('center_axis',(0.734238830876792,-8.99183234042744E-17,
-0.678891257295808));
#47910=DIRECTION('ref_axis',(0.678891257295807,3.46311205996404E-31,0.734238830876791));
#47911=DIRECTION('',(0.734238830876791,0.,-0.678891257295807));
#47912=DIRECTION('center_axis',(-0.678891257295808,8.31402005216763E-17,
-0.734238830876792));
#47913=DIRECTION('ref_axis',(-0.734238830876792,-5.02124004685594E-34,0.678891257295808));
#47914=DIRECTION('',(0.734238830876791,-1.7529794737095E-16,-0.678891257295807));
#47915=DIRECTION('',(0.,1.,0.));
#47916=DIRECTION('',(0.,-1.,0.));
#47917=DIRECTION('center_axis',(3.65737147181347E-17,1.,5.60477622923109E-17));
#47918=DIRECTION('ref_axis',(-0.837468181754969,0.,0.54648608815598));
#47919=DIRECTION('center_axis',(0.814436178114135,-9.97396658637165E-17,
0.580253144566095));
#47920=DIRECTION('ref_axis',(0.580253144566095,-1.05208313255741E-31,-0.814436178114135));
#47921=DIRECTION('center_axis',(1.22464679915E-16,1.,3.21507022015E-32));
#47922=DIRECTION('ref_axis',(1.,-1.22464679915E-16,-3.93732545414918E-48));
#47923=DIRECTION('center_axis',(0.54648608815598,-6.69252438638976E-17,
0.837468181754969));
#47924=DIRECTION('ref_axis',(0.837468181754969,1.49530298329546E-31,-0.54648608815598));
#47925=DIRECTION('center_axis',(1.,0.,0.));
#47926=DIRECTION('ref_axis',(0.,-1.,0.));
#47927=DIRECTION('center_axis',(-1.22464679915E-16,-1.,-2.46519032882E-32));
#47928=DIRECTION('ref_axis',(1.,-1.22464679915E-16,-3.01898744548495E-48));
#47929=DIRECTION('center_axis',(-1.224646799149E-16,-1.,1.07586726537792E-28));
#47930=DIRECTION('ref_axis',(-0.678891257295809,8.31402005216766E-17,-0.73423883087679));
#47931=DIRECTION('center_axis',(-1.22464679915E-16,-1.,-2.46519032882E-32));
#47932=DIRECTION('ref_axis',(1.,-1.22464679915E-16,-3.01898744548495E-48));
#47933=DIRECTION('',(0.,-1.,0.));
#47934=DIRECTION('center_axis',(1.22464679914909E-16,1.,-6.61121943250621E-29));
#47935=DIRECTION('ref_axis',(-0.809156716779487,9.90931183213597E-17,-0.587592892818354));
#47936=DIRECTION('',(0.,-1.,0.));
#47937=DIRECTION('center_axis',(1.22464679915E-16,1.,2.46519032882E-32));
#47938=DIRECTION('ref_axis',(1.,-1.22464679915E-16,-3.01898744548495E-48));
#47939=DIRECTION('center_axis',(0.734238830876792,-8.99183234042744E-17,
-0.678891257295808));
#47940=DIRECTION('ref_axis',(0.678891257295807,3.46311205996404E-31,0.734238830876791));
#47941=DIRECTION('',(-0.734238830876791,0.,0.678891257295807));
#47942=DIRECTION('center_axis',(-0.734238830876792,8.99183234042744E-17,
0.678891257295808));
#47943=DIRECTION('ref_axis',(0.678891257295808,1.51038693775819E-31,0.734238830876792));
#47944=DIRECTION('center_axis',(0.,0.,1.));
#47945=DIRECTION('ref_axis',(1.,0.,0.));
#47946=DIRECTION('center_axis',(-1.22464679915E-16,-1.,-3.69778549322E-32));
#47947=DIRECTION('ref_axis',(1.,-1.22464679915E-16,-4.52848116821518E-48));
#47948=DIRECTION('center_axis',(1.224646799149E-16,1.,-1.07586726537792E-28));
#47949=DIRECTION('ref_axis',(0.678891257295809,-8.31402005216765E-17,0.73423883087679));
#47950=DIRECTION('center_axis',(-1.22464679915E-16,-1.,-2.46519032882E-32));
#47951=DIRECTION('ref_axis',(1.,-1.22464679915E-16,-3.01898744548495E-48));
#47952=DIRECTION('',(0.,-1.,0.));
#47953=DIRECTION('center_axis',(-0.678891257295808,8.31402005216763E-17,
-0.734238830876792));
#47954=DIRECTION('ref_axis',(-0.734238830876792,-5.02124004685594E-34,0.678891257295808));
#47955=DIRECTION('',(0.,-1.,0.));
#47956=DIRECTION('',(-0.734238830876791,1.47705801254958E-16,0.678891257295807));
#47957=DIRECTION('center_axis',(1.22464679915E-16,1.,3.21507022015E-32));
#47958=DIRECTION('ref_axis',(1.,-1.22464679915E-16,0.));
#47959=DIRECTION('',(0.734238830876791,0.,0.678891257295807));
#47960=DIRECTION('center_axis',(1.22464679915E-16,1.,2.46519032882E-32));
#47961=DIRECTION('ref_axis',(1.,-1.22464679915E-16,-3.01898744548495E-48));
#47962=DIRECTION('',(-0.734238830876791,0.,-0.678891257295807));
#47963=DIRECTION('center_axis',(-1.22464679915E-16,-1.,-2.46519032882E-32));
#47964=DIRECTION('ref_axis',(1.,-1.22464679915E-16,2.53931026341659E-48));
#47965=DIRECTION('center_axis',(-1.22464679915E-16,-1.,-2.46519032882E-32));
#47966=DIRECTION('ref_axis',(1.,-1.22464679915E-16,-3.01898744548495E-48));
#47967=DIRECTION('center_axis',(-0.734238830876792,8.99183234039869E-17,
-0.678891257295808));
#47968=DIRECTION('ref_axis',(-6.60215246505446E-17,-1.,-6.10447636296637E-17));
#47969=DIRECTION('center_axis',(-0.734238830876792,8.99183234042744E-17,
-0.678891257295808));
#47970=DIRECTION('ref_axis',(0.678891257295807,3.46311205996404E-31,-0.734238830876791));
#47971=DIRECTION('',(-0.734238830876791,0.,-0.678891257295807));
#47972=DIRECTION('center_axis',(-0.678891257295808,8.31402005216763E-17,
0.734238830876792));
#47973=DIRECTION('ref_axis',(1.22464679914784E-16,1.,1.83887638005312E-34));
#47974=DIRECTION('',(-0.734238830876791,1.47829617289958E-16,-0.678891257295807));
#47975=DIRECTION('',(0.,1.,0.));
#47976=DIRECTION('',(0.,1.,0.));
#47977=DIRECTION('center_axis',(0.,0.,1.));
#47978=DIRECTION('ref_axis',(1.,0.,0.));
#47979=DIRECTION('center_axis',(0.814436178114135,-9.97396658637165E-17,
-0.580253144566095));
#47980=DIRECTION('ref_axis',(0.580253144566095,-3.4207048899363E-31,0.814436178114135));
#47981=DIRECTION('center_axis',(-1.22464679915E-16,-1.,-3.69778549322E-32));
#47982=DIRECTION('ref_axis',(1.,-1.22464679915E-16,-4.52848116821518E-48));
#47983=DIRECTION('center_axis',(1.22464679914972E-16,1.,-3.85870763968785E-29));
#47984=DIRECTION('ref_axis',(-0.580253144566094,7.10605156189115E-17,-0.814436178114135));
#47985=DIRECTION('center_axis',(-1.22464679915E-16,-1.,-3.69778549322E-32));
#47986=DIRECTION('ref_axis',(1.,-1.22464679915E-16,-4.52848116821518E-48));
#47987=DIRECTION('',(0.,1.,0.));
#47988=DIRECTION('center_axis',(1.22464679914909E-16,1.,-6.61121943250621E-29));
#47989=DIRECTION('ref_axis',(0.721410252528561,-8.83472756631981E-17,0.692507940421391));
#47990=DIRECTION('center_axis',(1.22464679915E-16,1.,2.46519032882E-32));
#47991=DIRECTION('ref_axis',(1.,-1.22464679915E-16,-3.01898744548495E-48));
#47992=DIRECTION('',(0.,-1.,0.));
#47993=DIRECTION('center_axis',(8.12315922726109E-17,1.,-5.78742547555248E-17));
#47994=DIRECTION('ref_axis',(0.580253144566096,0.,0.814436178114134));
#47995=DIRECTION('center_axis',(0.54648608815598,-6.69252438638976E-17,
-0.837468181754969));
#47996=DIRECTION('ref_axis',(0.837468181754969,1.49530298329546E-31,0.54648608815598));
#47997=DIRECTION('center_axis',(-0.734238830876792,8.99183234042744E-17,
-0.678891257295808));
#47998=DIRECTION('ref_axis',(0.678891257295807,3.46311205996404E-31,-0.734238830876791));
#47999=DIRECTION('',(0.734238830876791,0.,0.678891257295807));
#48000=DIRECTION('center_axis',(0.734238830876792,-8.99183234042744E-17,
0.678891257295808));
#48001=DIRECTION('ref_axis',(0.678891257295808,1.72414837744489E-31,-0.734238830876792));
#48002=DIRECTION('center_axis',(1.,0.,0.));
#48003=DIRECTION('ref_axis',(0.,-1.,0.));
#48004=DIRECTION('center_axis',(-1.22464679915E-16,-1.,-2.46519032882E-32));
#48005=DIRECTION('ref_axis',(1.,-1.22464679915E-16,-3.01898744548495E-48));
#48006=DIRECTION('center_axis',(1.224646799149E-16,1.,1.07603845915075E-28));
#48007=DIRECTION('ref_axis',(0.678891257295809,-8.31402005216765E-17,-0.73423883087679));
#48008=DIRECTION('center_axis',(-1.22464679915E-16,-1.,-2.46519032882E-32));
#48009=DIRECTION('ref_axis',(1.,-1.22464679915E-16,-3.01898744548495E-48));
#48010=DIRECTION('',(0.,-1.,0.));
#48011=DIRECTION('center_axis',(-0.678891257295808,8.31402005216763E-17,
0.734238830876792));
#48012=DIRECTION('ref_axis',(1.22464679914784E-16,1.,1.83887638005312E-34));
#48013=DIRECTION('',(0.,-1.,0.));
#48014=DIRECTION('',(0.734238830876791,-1.7634971726895E-16,0.678891257295807));
#48015=DIRECTION('center_axis',(1.,-1.22464679915E-16,2.44929359829E-16));
#48016=DIRECTION('ref_axis',(-2.44929359829E-16,0.,1.));
#48017=DIRECTION('',(2.54245135096E-16,0.,-1.));
#48018=DIRECTION('',(-1.4098070154E-16,-1.,0.));
#48019=DIRECTION('',(3.06496402452E-16,0.,-1.));
#48020=DIRECTION('',(2.04649405461E-16,1.,0.));
#48021=DIRECTION('center_axis',(-2.44929359829E-16,5.34329236504435E-33,
1.));
#48022=DIRECTION('ref_axis',(-1.3087291783495E-48,-1.,5.34329236504435E-33));
#48023=DIRECTION('',(2.04893992976E-16,0.,-1.));
#48024=DIRECTION('center_axis',(3.01898744547E-48,2.46519032882E-32,-1.));
#48025=DIRECTION('ref_axis',(1.,-7.44237865340164E-80,3.01898744547E-48));
#48026=DIRECTION('center_axis',(1.22464679915E-16,1.,3.21507022015E-32));
#48027=DIRECTION('ref_axis',(1.,-1.22464679915E-16,0.));
#48028=DIRECTION('',(-3.06496402452E-16,0.,1.));
#48029=DIRECTION('center_axis',(-1.22464679915E-16,-1.,-3.08148791102E-32));
#48030=DIRECTION('ref_axis',(1.,-1.22464679915E-16,-3.77373430685006E-48));
#48031=DIRECTION('center_axis',(-1.22464679915E-16,-1.,-3.08148791102E-32));
#48032=DIRECTION('ref_axis',(1.,-1.22464679915E-16,-3.77373430685006E-48));
#48033=DIRECTION('center_axis',(-1.22464679915E-16,-1.,-2.46519032882E-32));
#48034=DIRECTION('ref_axis',(1.,-1.22464679915E-16,-3.01898744548495E-48));
#48035=DIRECTION('center_axis',(1.22464679915E-16,1.,2.46519032882E-32));
#48036=DIRECTION('ref_axis',(1.,-1.22464679915E-16,2.36438383255719E-48));
#48037=DIRECTION('center_axis',(1.22464679915E-16,1.,3.38963670212E-32));
#48038=DIRECTION('ref_axis',(1.,-1.22464679915E-16,-4.15110773753262E-48));
#48039=DIRECTION('center_axis',(1.22464679915E-16,1.,3.08148791102E-32));
#48040=DIRECTION('ref_axis',(1.,-1.22464679915E-16,2.9554797906917E-48));
#48041=DIRECTION('center_axis',(1.22464679914907E-16,1.,1.86840883671487E-28));
#48042=DIRECTION('ref_axis',(-0.446669893168924,5.47012854943908E-17,0.894698835662851));
#48043=DIRECTION('center_axis',(1.22464679915E-16,1.,3.21507022015E-32));
#48044=DIRECTION('ref_axis',(1.,-1.22464679915E-16,-3.93732545414918E-48));
#48045=DIRECTION('center_axis',(1.22464679915E-16,1.,3.08148791102E-32));
#48046=DIRECTION('ref_axis',(1.,-1.22464679915E-16,-3.77373430685006E-48));
#48047=DIRECTION('',(0.,1.,0.));
#48048=DIRECTION('center_axis',(1.,0.,0.));
#48049=DIRECTION('ref_axis',(0.,-1.,0.));
#48050=DIRECTION('center_axis',(0.894698835662851,-1.09569006529982E-16,
0.446669893168925));
#48051=DIRECTION('ref_axis',(0.446669893168925,-6.79741207737406E-32,-0.894698835662851));
#48052=DIRECTION('center_axis',(9.80312625669243E-17,1.,4.89411764412796E-17));
#48053=DIRECTION('ref_axis',(0.446669893168925,0.,-0.894698835662851));
#48054=DIRECTION('center_axis',(-1.22464679915E-16,-1.,-3.21507022015E-32));
#48055=DIRECTION('ref_axis',(1.,-1.22464679915E-16,-3.93732545414918E-48));
#48056=DIRECTION('center_axis',(0.965607221472844,-1.18252779300981E-16,
0.260005180408957));
#48057=DIRECTION('ref_axis',(0.260005180408957,3.6319060404761E-32,-0.965607221472844));
#48058=DIRECTION('center_axis',(1.22464679914936E-16,1.,1.40353954282933E-28));
#48059=DIRECTION('ref_axis',(0.35511183407264,-4.34886570935806E-17,-0.934823825809744));
#48060=DIRECTION('',(1.43023900113E-16,1.,0.));
#48061=DIRECTION('center_axis',(-1.22464679915E-16,-1.,-2.46519032882E-32));
#48062=DIRECTION('ref_axis',(1.,-1.22464679915E-16,-3.01898744548495E-48));
#48063=DIRECTION('center_axis',(1.14185737652554E-16,1.,3.07463352160911E-17));
#48064=DIRECTION('ref_axis',(0.260005180408958,0.,-0.965607221472844));
#48065=DIRECTION('center_axis',(-1.22464679915E-16,-1.,-3.08148791102E-32));
#48066=DIRECTION('ref_axis',(1.,-1.22464679915E-16,-3.77373430685006E-48));
#48067=DIRECTION('center_axis',(0.965607221472844,-1.18252779300981E-16,
-0.260005180408957));
#48068=DIRECTION('ref_axis',(0.260005180408957,3.6319060404761E-32,0.965607221472844));
#48069=DIRECTION('center_axis',(1.22464679915E-16,1.,3.03685191950031E-32));
#48070=DIRECTION('ref_axis',(-6.0392731067552E-15,7.69966167133047E-31,
-1.));
#48071=DIRECTION('',(0.,1.,0.));
#48072=DIRECTION('center_axis',(-1.22464679915E-16,-1.,-3.08148791102E-32));
#48073=DIRECTION('ref_axis',(1.,-1.22464679915E-16,-3.77373430685006E-48));
#48074=DIRECTION('center_axis',(1.14185737652555E-16,1.,-3.07463352160911E-17));
#48075=DIRECTION('ref_axis',(-0.260005180408958,0.,-0.965607221472844));
#48076=DIRECTION('center_axis',(-1.22464679915E-16,-1.,-3.21507022015E-32));
#48077=DIRECTION('ref_axis',(1.,-1.22464679915E-16,-3.93732545414918E-48));
#48078=DIRECTION('center_axis',(0.894698835662851,-1.09569006529982E-16,
-0.446669893168925));
#48079=DIRECTION('ref_axis',(0.446669893168925,-6.79741207737406E-32,0.894698835662851));
#48080=DIRECTION('center_axis',(1.22464679914936E-16,1.,-1.40336501664893E-28));
#48081=DIRECTION('ref_axis',(-0.35511183407264,4.34886570935806E-17,-0.934823825809744));
#48082=DIRECTION('',(-2.04649405461E-16,-1.,0.));
#48083=DIRECTION('center_axis',(-1.22464679915E-16,-1.,-3.08148791102E-32));
#48084=DIRECTION('ref_axis',(1.,-1.22464679915E-16,-3.77373430685006E-48));
#48085=DIRECTION('center_axis',(-2.44929359829E-16,5.34329236508E-33,1.));
#48086=DIRECTION('ref_axis',(-1.,-1.30872917835823E-48,-2.44929359829E-16));
#48087=DIRECTION('',(-2.71043176004E-16,0.,1.));
#48088=DIRECTION('center_axis',(1.15648231732E-16,-3.88147269699E-32,1.));
#48089=DIRECTION('ref_axis',(1.,4.48885453922931E-48,-1.15648231732E-16));
#48090=DIRECTION('center_axis',(1.,0.,0.));
#48091=DIRECTION('ref_axis',(0.,-1.,0.));
#48092=DIRECTION('center_axis',(1.22464679915E-16,1.,3.21507022015E-32));
#48093=DIRECTION('ref_axis',(1.,-1.22464679915E-16,-3.93732545414918E-48));
#48094=DIRECTION('center_axis',(1.22464679915E-16,1.,3.21507022015E-32));
#48095=DIRECTION('ref_axis',(-1.,1.22464679915E-16,3.93732545414918E-48));
#48096=DIRECTION('center_axis',(1.22464679915E-16,1.,3.08148791102E-32));
#48097=DIRECTION('ref_axis',(1.,-1.22464679915E-16,-3.77373430685006E-48));
#48098=DIRECTION('',(-1.43023900113E-16,-1.,0.));
#48099=DIRECTION('center_axis',(1.,-1.22464679915E-16,2.44929359829E-16));
#48100=DIRECTION('ref_axis',(-2.44929359829E-16,0.,1.));
#48101=DIRECTION('',(1.4098070154E-16,1.,0.));
#48102=DIRECTION('',(-2.54245135096E-16,0.,1.));
#48103=DIRECTION('center_axis',(-1.22464679915E-16,-1.,-3.21507022015E-32));
#48104=DIRECTION('ref_axis',(-1.,1.22464679915E-16,0.));
#48105=DIRECTION('center_axis',(-1.22464679915E-16,-1.,-3.21507022015E-32));
#48106=DIRECTION('ref_axis',(1.,-1.22464679915E-16,-3.93732545414918E-48));
#48107=DIRECTION('center_axis',(1.22464679915E-16,1.,3.38963670212E-32));
#48108=DIRECTION('ref_axis',(1.,-1.22464679915E-16,-4.15110773753262E-48));
#48109=DIRECTION('center_axis',(-1.22464679915E-16,-1.,-3.21507022015E-32));
#48110=DIRECTION('ref_axis',(1.,-1.22464679915E-16,-3.93732545414918E-48));
#48111=DIRECTION('center_axis',(1.22464679915E-16,1.,3.08148791102E-32));
#48112=DIRECTION('ref_axis',(1.,-1.22464679915E-16,-3.77373430685006E-48));
#48113=DIRECTION('center_axis',(-1.22464679915E-16,-1.,-3.21507022015E-32));
#48114=DIRECTION('ref_axis',(1.,-1.22464679915E-16,-3.93732545414918E-48));
#48115=DIRECTION('center_axis',(1.22464679915E-16,1.,3.69778549322E-32));
#48116=DIRECTION('ref_axis',(1.,-1.22464679915E-16,-4.52848116821518E-48));
#48117=DIRECTION('center_axis',(0.734238830876792,-8.99183234039869E-17,
-0.678891257295808));
#48118=DIRECTION('ref_axis',(2.09848214201023E-17,1.,-1.09753148030108E-16));
#48119=DIRECTION('center_axis',(0.734238830876792,-2.0982535965894E-15,
-0.678891257295808));
#48120=DIRECTION('ref_axis',(0.678891257295807,8.02543484770833E-30,0.734238830876791));
#48121=DIRECTION('center_axis',(0.734238830876792,-8.99183234042744E-17,
-0.678891257295808));
#48122=DIRECTION('ref_axis',(0.678891257295808,1.72414837744489E-31,0.734238830876792));
#48123=DIRECTION('',(0.734238830876791,0.,-0.678891257295807));
#48124=DIRECTION('center_axis',(-6.60215246509141E-17,-1.,6.10447636300053E-17));
#48125=DIRECTION('ref_axis',(-0.678891257295808,0.,-0.734238830876791));
#48126=DIRECTION('center_axis',(0.54648608815598,-6.69252438638976E-17,
0.837468181754969));
#48127=DIRECTION('ref_axis',(0.837468181754969,-2.14539310633749E-32,-0.54648608815598));
#48128=DIRECTION('center_axis',(-1.22464679915E-16,-1.,-3.21507022015E-32));
#48129=DIRECTION('ref_axis',(1.,-1.22464679915E-16,-3.93732545414918E-48));
#48130=DIRECTION('center_axis',(-8.12315922726109E-17,-1.,-5.78742547555248E-17));
#48131=DIRECTION('ref_axis',(-0.580253144566096,0.,0.814436178114134));
#48132=DIRECTION('center_axis',(0.814436178114135,-9.97396658637165E-17,
0.580253144566095));
#48133=DIRECTION('ref_axis',(0.580253144566095,-1.05208313255741E-31,-0.814436178114135));
#48134=DIRECTION('center_axis',(1.22464679915E-16,1.,3.21507022015E-32));
#48135=DIRECTION('ref_axis',(1.,-1.22464679915E-16,-3.93732545414918E-48));
#48136=DIRECTION('center_axis',(-8.12315922726109E-17,-1.,-5.78742547555248E-17));
#48137=DIRECTION('ref_axis',(0.580253144566096,0.,-0.814436178114134));
#48138=DIRECTION('center_axis',(-0.734238830876792,8.99183234042744E-17,
0.678891257295808));
#48139=DIRECTION('ref_axis',(0.678891257295808,1.51038693775819E-31,0.734238830876792));
#48140=DIRECTION('center_axis',(-1.22464679915E-16,-1.,-3.21507022015E-32));
#48141=DIRECTION('ref_axis',(1.,-1.22464679915E-16,-3.93732545414918E-48));
#48142=DIRECTION('center_axis',(0.734238830876792,-8.99183234042744E-17,
-0.678891257295808));
#48143=DIRECTION('ref_axis',(-0.678891257295808,1.09298769049165E-33,-0.734238830876792));
#48144=DIRECTION('center_axis',(-0.734238830876792,-3.99271497926887E-15,
0.678891257295808));
#48145=DIRECTION('ref_axis',(0.678891257295807,-1.5084889012382E-29,0.734238830876791));
#48146=DIRECTION('',(-0.734238830876791,0.,0.678891257295807));
#48147=DIRECTION('center_axis',(-0.734238830876792,8.99183234039869E-17,
-0.678891257295808));
#48148=DIRECTION('ref_axis',(6.60215246505446E-17,1.,6.10447636296637E-17));
#48149=DIRECTION('center_axis',(-0.734238830876792,2.56033960610927E-18,
-0.678891257295808));
#48150=DIRECTION('ref_axis',(0.678891257295807,9.76887763626404E-33,-0.734238830876791));
#48151=DIRECTION('center_axis',(-0.734238830876792,8.99183234042744E-17,
-0.678891257295808));
#48152=DIRECTION('ref_axis',(0.678891257295808,1.51038693775819E-31,-0.734238830876792));
#48153=DIRECTION('',(-0.734238830876791,0.,-0.678891257295807));
#48154=DIRECTION('center_axis',(-6.60215246509141E-17,-1.,-6.10447636300053E-17));
#48155=DIRECTION('ref_axis',(-0.678891257295808,0.,0.734238830876791));
#48156=DIRECTION('center_axis',(-1.22464679915E-16,-1.,-3.21507022015E-32));
#48157=DIRECTION('ref_axis',(1.,-1.22464679915E-16,-3.93732545414918E-48));
#48158=DIRECTION('center_axis',(-3.65737147181347E-17,-1.,5.60477622923109E-17));
#48159=DIRECTION('ref_axis',(-0.83746818175497,0.,-0.54648608815598));
#48160=DIRECTION('center_axis',(0.734238830876792,-8.99183234042744E-17,
0.678891257295808));
#48161=DIRECTION('ref_axis',(0.678891257295808,1.72414837744489E-31,-0.734238830876792));
#48162=DIRECTION('center_axis',(-1.22464679915E-16,-1.,-3.21507022015E-32));
#48163=DIRECTION('ref_axis',(1.,-1.22464679915E-16,-3.93732545414918E-48));
#48164=DIRECTION('center_axis',(-0.734238830876792,8.99183234042744E-17,
-0.678891257295808));
#48165=DIRECTION('ref_axis',(-0.678891257295808,1.01431800150836E-32,0.734238830876792));
#48166=DIRECTION('center_axis',(0.734238830876792,1.02275665268971E-14,
0.678891257295808));
#48167=DIRECTION('ref_axis',(0.678891257295807,-1.15648231731787E-14,-0.734238830876791));
#48168=DIRECTION('',(0.734238830876791,0.,0.678891257295807));
#48169=DIRECTION('center_axis',(-2.44929359829E-16,5.34329236504435E-33,
1.));
#48170=DIRECTION('ref_axis',(1.3087291783495E-48,1.,-5.34329236504435E-33));
#48171=DIRECTION('center_axis',(3.20552409216E-15,-3.67911578618E-31,-1.));
#48172=DIRECTION('ref_axis',(1.,1.15641341524065E-46,3.20552409216E-15));
#48173=DIRECTION('',(4.25315706605E-16,0.,-1.));
#48174=DIRECTION('center_axis',(2.44929359829E-16,-9.25185853854E-17,-1.));
#48175=DIRECTION('ref_axis',(1.,2.26605178907307E-32,2.44929359829E-16));
#48176=DIRECTION('center_axis',(-1.00043346337309E-45,-1.,3.37916382964629E-31));
#48177=DIRECTION('ref_axis',(1.,0.,2.96059473233375E-15));
#48178=DIRECTION('center_axis',(0.894698835662851,-1.09569006529982E-16,
0.446669893168925));
#48179=DIRECTION('ref_axis',(0.446669893168925,7.79859429427442E-32,-0.894698835662851));
#48180=DIRECTION('center_axis',(1.22464679915E-16,1.,3.21507022015E-32));
#48181=DIRECTION('ref_axis',(1.,-1.22464679915E-16,-3.93732545414918E-48));
#48182=DIRECTION('center_axis',(-1.14185737652555E-16,-1.,-3.07463352160911E-17));
#48183=DIRECTION('ref_axis',(0.260005180408958,0.,-0.965607221472844));
#48184=DIRECTION('center_axis',(0.965607221472844,-1.18252779300981E-16,
0.260005180408957));
#48185=DIRECTION('ref_axis',(0.260005180408957,3.6319060404761E-32,-0.965607221472844));
#48186=DIRECTION('center_axis',(-1.22464679915E-16,-1.,-3.21507022015E-32));
#48187=DIRECTION('ref_axis',(1.,-1.22464679915E-16,-3.93732545414918E-48));
#48188=DIRECTION('center_axis',(-1.14185737652555E-16,-1.,3.07463352160911E-17));
#48189=DIRECTION('ref_axis',(-0.260005180408958,0.,-0.965607221472844));
#48190=DIRECTION('center_axis',(0.965607221472844,-1.18252779300981E-16,
-0.260005180408957));
#48191=DIRECTION('ref_axis',(0.260005180408957,3.6319060404761E-32,0.965607221472844));
#48192=DIRECTION('center_axis',(-1.22464679915E-16,-1.,-3.21507022015E-32));
#48193=DIRECTION('ref_axis',(1.,-1.22464679915E-16,-3.93732545414918E-48));
#48194=DIRECTION('center_axis',(-9.80312625669243E-17,-1.,4.89411764412795E-17));
#48195=DIRECTION('ref_axis',(-0.446669893168925,0.,-0.894698835662851));
#48196=DIRECTION('center_axis',(0.894698835662851,-1.09569006529982E-16,
-0.446669893168925));
#48197=DIRECTION('ref_axis',(0.446669893168925,7.79859429427442E-32,0.894698835662851));
#48198=DIRECTION('center_axis',(-1.22464679915E-16,-1.,-3.21507022015E-32));
#48199=DIRECTION('ref_axis',(1.,-1.22464679915E-16,-3.93732545414918E-48));
#48200=DIRECTION('center_axis',(-9.80312625669243E-17,-1.,4.89411764412795E-17));
#48201=DIRECTION('ref_axis',(0.446669893168926,0.,0.894698835662851));
#48202=DIRECTION('center_axis',(-2.44929359829E-16,5.34329236508E-33,1.));
#48203=DIRECTION('ref_axis',(1.,1.30872917835823E-48,2.44929359829E-16));
#48204=DIRECTION('center_axis',(1.22464679915E-16,1.,3.21507022015E-32));
#48205=DIRECTION('ref_axis',(1.,-1.22464679915E-16,-3.93732545414918E-48));
#48206=DIRECTION('center_axis',(-2.44929359829E-16,5.34329236508E-33,1.));
#48207=DIRECTION('ref_axis',(1.,1.30872917835823E-48,2.44929359829E-16));
#48208=DIRECTION('center_axis',(5.67626010484E-15,-1.38777878078E-16,1.));
#48209=DIRECTION('ref_axis',(1.,-1.47314773920115E-32,-5.67626010484E-15));
#48210=DIRECTION('',(-4.25315706605E-16,0.,1.));
#48211=DIRECTION('center_axis',(-1.22464679915E-16,-1.,-3.21507022015E-32));
#48212=DIRECTION('ref_axis',(-1.,1.22464679915E-16,0.));
#48213=DIRECTION('center_axis',(-1.22464679915E-16,-1.,-3.08148791102E-32));
#48214=DIRECTION('ref_axis',(1.,-1.22464679915E-16,2.9554797906917E-48));
#48215=DIRECTION('center_axis',(-1.22464679915E-16,-1.,-3.08148791102E-32));
#48216=DIRECTION('ref_axis',(1.,-1.22464679915E-16,2.9554797906917E-48));
#48217=DIRECTION('center_axis',(-1.22464679915E-16,-1.,-2.46519032882E-32));
#48218=DIRECTION('ref_axis',(1.,-1.22464679915E-16,2.53931026341659E-48));
#48219=DIRECTION('center_axis',(0.221508968488806,0.953407602538901,0.204811426195051));
#48220=DIRECTION('ref_axis',(0.700028883437118,-0.301685172690054,0.647260086003111));
#48221=DIRECTION('center_axis',(-1.22464679915E-16,-1.,-2.46519032882E-32));
#48222=DIRECTION('ref_axis',(1.,-1.22464679915E-16,-3.01898744548495E-48));
#48223=DIRECTION('center_axis',(0.184321578630023,-2.25728831283027E-17,
-0.982865990688118));
#48224=DIRECTION('ref_axis',(0.982865990688118,3.73386811100911E-32,0.184321578630023));
#48225=DIRECTION('center_axis',(-0.678891257295897,3.86265093984168E-14,
0.734238830876709));
#48226=DIRECTION('ref_axis',(-0.70002888343712,0.301685172690054,-0.647260086003109));
#48227=DIRECTION('center_axis',(0.,0.235800057020902,-0.971801591431574));
#48228=DIRECTION('ref_axis',(0.,0.971801591431575,0.235800057020898));
#48229=DIRECTION('center_axis',(-0.905552945157821,1.10898251574978E-16,
-0.424233265451916));
#48230=DIRECTION('ref_axis',(0.424233265451916,2.2812757295719E-31,-0.905552945157821));
#48231=DIRECTION('center_axis',(-1.22464679915E-16,-1.,-3.08148791102E-32));
#48232=DIRECTION('ref_axis',(1.,-1.22464679915E-16,-3.77373430685006E-48));
#48233=DIRECTION('center_axis',(-1.,6.29350163966441E-17,-2.59373767181107E-16));
#48234=DIRECTION('ref_axis',(0.,-0.971801591431574,-0.235800057020901));
#48235=DIRECTION('center_axis',(-1.22464679915E-16,-1.,-3.08148791102E-32));
#48236=DIRECTION('ref_axis',(1.,-1.22464679915E-16,-3.77373430685006E-48));
#48237=DIRECTION('center_axis',(-1.16760731574493E-16,-1.,-2.58069211860055E-17));
#48238=DIRECTION('ref_axis',(0.215815367394074,0.,-0.976434189895336));
#48239=DIRECTION('center_axis',(-1.22464679915E-16,-1.,-3.21507022015E-32));
#48240=DIRECTION('ref_axis',(1.,-1.22464679915E-16,2.95348236287722E-48));
#48241=DIRECTION('center_axis',(-1.22464679915E-16,-1.,-2.46519032882E-32));
#48242=DIRECTION('ref_axis',(1.,-1.22464679915E-16,-3.01898744548495E-48));
#48243=DIRECTION('center_axis',(-0.201250650785258,-0.315250304640726,0.927424078284816));
#48244=DIRECTION('ref_axis',(-0.244245415585181,0.93304050163127,0.264158284521404));
#48245=DIRECTION('center_axis',(1.224646799149E-16,1.,1.07603845915075E-28));
#48246=DIRECTION('ref_axis',(-0.67889125729581,8.31402005216767E-17,0.734238830876789));
#48247=DIRECTION('',(0.,-1.,0.));
#48248=DIRECTION('center_axis',(-1.22464679915E-16,-1.,-3.08148791102001E-32));
#48249=DIRECTION('ref_axis',(-1.,1.22464679915E-16,5.78241158658936E-15));
#48250=DIRECTION('',(-9.55030558817E-17,-1.,0.));
#48251=DIRECTION('center_axis',(-0.922303035444809,-6.8218782867173E-7,
-0.386467477038916));
#48252=DIRECTION('ref_axis',(-0.273271953394989,0.707112642513919,0.652161138281536));
#48253=DIRECTION('center_axis',(1.04173678864568E-16,1.,4.36513558728617E-17));
#48254=DIRECTION('ref_axis',(0.386467796953067,0.,-0.922302901393161));
#48255=DIRECTION('center_axis',(1.22464679915E-16,1.,3.21507022015E-32));
#48256=DIRECTION('ref_axis',(1.,-1.22464679915E-16,2.95348236287722E-48));
#48257=DIRECTION('center_axis',(-0.976434189895336,1.19578700523041E-16,
-0.215815367394074));
#48258=DIRECTION('ref_axis',(0.215815367394074,2.78959734683971E-32,-0.976434189895336));
#48259=DIRECTION('center_axis',(-1.22464679914995E-16,-1.,-2.84643200354157E-29));
#48260=DIRECTION('ref_axis',(0.175818770215043,-2.15315894174053E-17,-0.984422551570244));
#48261=DIRECTION('',(0.,-1.,0.));
#48262=DIRECTION('',(-1.27905878413E-16,-1.,0.));
#48263=DIRECTION('center_axis',(1.16760731574493E-16,1.,2.58069211860055E-17));
#48264=DIRECTION('ref_axis',(0.215815367394074,0.,-0.976434189895336));
#48265=DIRECTION('center_axis',(1.22464679915E-16,1.,3.08148791102E-32));
#48266=DIRECTION('ref_axis',(1.,-1.22464679915E-16,-3.77373430685006E-48));
#48267=DIRECTION('center_axis',(-0.976434189895336,1.19578700523041E-16,
0.215815367394074));
#48268=DIRECTION('ref_axis',(0.215815367394074,2.78959734683971E-32,0.976434189895336));
#48269=DIRECTION('center_axis',(1.22464679914969E-16,1.,1.40937670198757E-28));
#48270=DIRECTION('ref_axis',(0.215815367394074,-2.64297598885091E-17,-0.976434189895336));
#48271=DIRECTION('',(-9.55030558817E-17,-1.,0.));
#48272=DIRECTION('center_axis',(-0.716038439225428,0.221273058165028,0.662062827292024));
#48273=DIRECTION('ref_axis',(0.162467271531971,0.97521189170882,-0.150220344662972));
#48274=DIRECTION('center_axis',(1.22464679915E-16,1.,2.46519032882E-32));
#48275=DIRECTION('ref_axis',(1.,-1.22464679915E-16,-3.01898744548495E-48));
#48276=DIRECTION('center_axis',(0.678891257295725,-4.93644477147132E-13,
0.734238830876867));
#48277=DIRECTION('ref_axis',(-0.162467271531966,-0.97521189170882,0.150220344662973));
#48278=DIRECTION('center_axis',(1.22464679915E-16,1.,2.46519032882E-32));
#48279=DIRECTION('ref_axis',(1.,-1.22464679915E-16,-3.01898744548495E-48));
#48280=DIRECTION('center_axis',(-0.184321578630023,2.25728831283027E-17,
-0.982865990688118));
#48281=DIRECTION('ref_axis',(0.982865990688118,3.73386811100911E-32,-0.184321578630023));
#48282=DIRECTION('center_axis',(-1.48029736616688E-15,0.958902687765847,
-0.283735150087956));
#48283=DIRECTION('ref_axis',(-7.4014868308344E-15,-0.28373515008795,-0.958902687765849));
#48284=DIRECTION('center_axis',(1.22464679915E-16,1.,2.46519032882E-32));
#48285=DIRECTION('ref_axis',(1.,-1.22464679915E-16,-3.01898744548495E-48));
#48286=DIRECTION('center_axis',(0.905552945157821,-1.10898251574978E-16,
-0.424233265451916));
#48287=DIRECTION('ref_axis',(0.424233265451916,8.51126007998586E-32,0.905552945157821));
#48288=DIRECTION('center_axis',(1.,-8.38443144529068E-16,-7.47061316104109E-15));
#48289=DIRECTION('ref_axis',(7.40148683083439E-15,0.28373515008795,0.958902687765849));
#48290=DIRECTION('center_axis',(-2.24037888703029E-16,-1.,2.20413632410453E-17));
#48291=DIRECTION('ref_axis',(-0.977255721664238,2.19472257881379E-16,0.212064269679052));
#48292=DIRECTION('center_axis',(-1.22464679915E-16,-1.,-3.21507022015E-32));
#48293=DIRECTION('ref_axis',(1.,-1.22464679915E-16,2.95348236287722E-48));
#48294=DIRECTION('center_axis',(-0.201250866957998,0.315250529579522,-0.927423954914086));
#48295=DIRECTION('ref_axis',(0.244245793120094,0.933040379819622,0.264158365699804));
#48296=DIRECTION('center_axis',(1.22464679915E-16,1.,2.46519032882E-32));
#48297=DIRECTION('ref_axis',(1.,-1.22464679915E-16,-3.01898744548495E-48));
#48298=DIRECTION('center_axis',(1.22464679915054E-16,1.,-1.00619139983431E-29));
#48299=DIRECTION('ref_axis',(-0.982865990688119,1.20366368949015E-16,0.184321578630021));
#48300=DIRECTION('',(1.91006111763E-16,1.,0.));
#48301=DIRECTION('center_axis',(1.16760731574493E-16,1.,-2.58069211860055E-17));
#48302=DIRECTION('ref_axis',(-0.215815367394074,0.,-0.976434189895336));
#48303=DIRECTION('center_axis',(1.22464679915E-16,1.,3.21507022015E-32));
#48304=DIRECTION('ref_axis',(1.,-1.22464679915E-16,2.95348236287722E-48));
#48305=DIRECTION('center_axis',(-0.922302870765176,-7.9241150460774E-8,
0.386467870046539));
#48306=DIRECTION('ref_axis',(-0.273273899979641,-0.707107039843237,-0.652166397320539));
#48307=DIRECTION('center_axis',(-1.22464679914968E-16,-1.,6.73818689876281E-29));
#48308=DIRECTION('ref_axis',(-0.424233265451918,5.19535910627899E-17,-0.905552945157821));
#48309=DIRECTION('',(9.55030558817E-17,1.,0.));
#48310=DIRECTION('center_axis',(-1.22464679914914E-16,-1.,-3.06469357969891E-29));
#48311=DIRECTION('ref_axis',(-0.941567095721782,1.15308712995973E-16,0.336825480410922));
#48312=DIRECTION('',(0.,-1.,0.));
#48313=DIRECTION('center_axis',(4.57540783324772E-17,1.,-5.92437580993829E-17));
#48314=DIRECTION('ref_axis',(0.791447785823259,0.,0.611236780892201));
#48315=DIRECTION('center_axis',(-0.299529302547155,-6.98450310923572E-8,
0.954087101325456));
#48316=DIRECTION('ref_axis',(-8.54331494437577E-8,0.999999999999995,4.63849662383584E-8));
#48317=DIRECTION('center_axis',(-0.611236780892201,7.48549167240244E-17,
0.791447785823259));
#48318=DIRECTION('ref_axis',(0.79144778582326,2.17825094235712E-31,0.611236780892201));
#48319=DIRECTION('center_axis',(-1.22464679915E-16,-1.,-3.69778549322E-32));
#48320=DIRECTION('ref_axis',(1.,-1.22464679915E-16,-4.52848116821518E-48));
#48321=DIRECTION('center_axis',(1.22464679914882E-16,1.,-9.11791729617953E-29));
#48322=DIRECTION('ref_axis',(0.79144778582326,-9.69243997601319E-17,0.611236780892201));
#48323=DIRECTION('',(-1.91006111763E-16,-1.,0.));
#48324=DIRECTION('center_axis',(1.09872665289959E-17,1.,3.49976006725472E-17));
#48325=DIRECTION('ref_axis',(-0.954087082104669,0.,0.299529363770896));
#48326=DIRECTION('center_axis',(-0.611236780892201,7.48549167240244E-17,
-0.791447785823259));
#48327=DIRECTION('ref_axis',(0.79144778582326,2.17825094235712E-31,-0.611236780892201));
#48328=DIRECTION('center_axis',(-0.299529300208521,-6.66484614947436E-8,
-0.954087102059654));
#48329=DIRECTION('ref_axis',(0.67464125064528,0.707106985515452,-0.211799183102824));
#48330=DIRECTION('center_axis',(-1.22464679915E-16,-1.,-3.38963670212E-32));
#48331=DIRECTION('ref_axis',(1.,-1.22464679915E-16,-4.15110773753262E-48));
#48332=DIRECTION('center_axis',(1.22464679914331E-16,1.,1.45106580954821E-28));
#48333=DIRECTION('ref_axis',(-0.977255721664238,1.19679309148029E-16,0.212064269679051));
#48334=DIRECTION('',(-1.91006111763E-16,-1.,0.));
#48335=DIRECTION('center_axis',(-0.194458884741274,0.964291220370907,0.17980040172582));
#48336=DIRECTION('ref_axis',(-0.708020058269897,-0.264844184975968,0.654648878996907));
#48337=DIRECTION('center_axis',(-1.22464679915E-16,-1.,-3.69778549322E-32));
#48338=DIRECTION('ref_axis',(1.,-1.22464679915E-16,-4.52848116821518E-48));
#48339=DIRECTION('center_axis',(0.823541624224482,-1.00854761407059E-16,
0.567255844544332));
#48340=DIRECTION('ref_axis',(0.567255844544332,2.21497266631789E-31,-0.823541624224482));
#48341=DIRECTION('center_axis',(-0.678891257295798,3.62846327058483E-15,
-0.7342388308768));
#48342=DIRECTION('ref_axis',(0.7080200582699,0.264844184975966,-0.654648878996905));
#48343=DIRECTION('center_axis',(0.710368265197812,0.252911675402861,0.656820076006183));
#48344=DIRECTION('ref_axis',(-0.185697572862959,0.967489371747782,-0.171699525298959));
#48345=DIRECTION('center_axis',(1.22464679915E-16,1.,3.69778549322E-32));
#48346=DIRECTION('ref_axis',(1.,-1.22464679915E-16,-4.52848116821518E-48));
#48347=DIRECTION('center_axis',(0.678891257295789,9.85612054934161E-14,
-0.734238830876809));
#48348=DIRECTION('ref_axis',(0.185697572862958,-0.967489371747782,0.171699525298964));
#48349=DIRECTION('center_axis',(1.22464679915E-16,1.,3.69778549322E-32));
#48350=DIRECTION('ref_axis',(1.,-1.22464679915E-16,-4.52848116821518E-48));
#48351=DIRECTION('center_axis',(-0.823541624224482,1.00854761407059E-16,
0.567255844544332));
#48352=DIRECTION('ref_axis',(0.567255844544332,2.21497266631789E-31,0.823541624224482));
#48353=DIRECTION('center_axis',(-4.57540783324772E-17,-1.,5.92437580993829E-17));
#48354=DIRECTION('ref_axis',(0.791447785823259,0.,0.611236780892201));
#48355=DIRECTION('center_axis',(-1.22464679915E-16,-1.,-3.21507022015E-32));
#48356=DIRECTION('ref_axis',(1.,-1.22464679915E-16,3.1731092887471E-48));
#48357=DIRECTION('center_axis',(4.57540783324772E-17,1.,5.92437580993829E-17));
#48358=DIRECTION('ref_axis',(-0.791447785823259,0.,0.611236780892201));
#48359=DIRECTION('center_axis',(-0.800318648295141,-2.90491584479981E-7,
-0.599574900401071));
#48360=DIRECTION('ref_axis',(-1.43841294430989E-7,0.999999999999947,-2.92495087409794E-7));
#48361=DIRECTION('center_axis',(-1.22464679915E-16,-1.,-3.21507022015E-32));
#48362=DIRECTION('ref_axis',(1.,-1.22464679915E-16,3.1731092887471E-48));
#48363=DIRECTION('center_axis',(1.224646799149E-16,1.,-1.07586726537792E-28));
#48364=DIRECTION('ref_axis',(-0.67889125729581,8.31402005216767E-17,-0.734238830876789));
#48365=DIRECTION('',(0.,-1.,0.));
#48366=DIRECTION('center_axis',(7.84398113463332E-17,1.,-5.8764805666941E-17));
#48367=DIRECTION('ref_axis',(0.599575127105149,0.,0.800318478455199));
#48368=DIRECTION('center_axis',(-0.80031675586116,2.87294455355871E-6,0.599577426425991));
#48369=DIRECTION('ref_axis',(0.424001176459416,-0.707044168099605,0.565960728953316));
#48370=DIRECTION('center_axis',(-1.22464679915E-16,-1.,-3.21507022015E-32));
#48371=DIRECTION('ref_axis',(1.,-1.22464679915E-16,3.1731092887471E-48));
#48372=DIRECTION('center_axis',(1.22464679914947E-16,1.,-7.73624659438748E-29));
#48373=DIRECTION('ref_axis',(0.567255844544333,-6.94688054319408E-17,0.82354162422448));
#48374=DIRECTION('',(0.,1.,0.));
#48375=DIRECTION('center_axis',(-1.22464679915E-16,-1.,-3.21507022014744E-32));
#48376=DIRECTION('ref_axis',(7.6571373978586E-16,-1.25923590250867E-31,
1.));
#95794=CARTESIAN_POINT('',(0.,0.,0.));
#95795=CARTESIAN_POINT('Origin',(-3.54162636048E-14,-23.4742356128,0.580061096522));
#95796=CARTESIAN_POINT('',(7.55300678542,-23.1742356128,11.1813685383));
#95797=CARTESIAN_POINT('',(10.9011091428,-23.1742356128,7.69353074443));
#95798=CARTESIAN_POINT('Origin',(-3.36841676743E-14,-23.1742356128,0.580061096522));
#95799=CARTESIAN_POINT('',(7.72708272879,-23.4742356128,11.4256993917));
#95800=CARTESIAN_POINT('Origin',(7.55300678542,-23.4742356128,11.1813685383));
#95801=CARTESIAN_POINT('',(11.1523495973,-23.4742356128,7.85747657088));
#95802=CARTESIAN_POINT('Origin',(-3.54162636048E-14,-23.4742356128,0.580061096522));
#95803=CARTESIAN_POINT('Origin',(10.9011091428,-23.4742356128,7.69353074443));
#95804=CARTESIAN_POINT('Origin',(-15.6588697715,-28.8242356128,14.965390674));
#95805=CARTESIAN_POINT('',(3.78111690148,-25.6742356128,-1.85483293631));
#95806=CARTESIAN_POINT('',(8.81393818057,-25.6742356128,7.09680280277));
#95807=CARTESIAN_POINT('Origin',(-15.6588697715,-25.6742356128,14.965390674));
#95808=CARTESIAN_POINT('',(3.78111690148,-32.4742356128,-1.85483293631));
#95809=CARTESIAN_POINT('',(3.78111690148,-28.8242356128,-1.85483293631));
#95810=CARTESIAN_POINT('',(8.81393818057,-32.4742356128,7.09680280277));
#95811=CARTESIAN_POINT('Origin',(-15.6588697715,-32.4742356128,14.965390674));
#95812=CARTESIAN_POINT('',(8.81393818057,-28.8242356128,7.09680280277));
#95813=CARTESIAN_POINT('Origin',(8.52833752869,-28.8242356128,7.18863018236));
#95814=CARTESIAN_POINT('',(8.74359670241,-25.6742356128,7.39758828372));
#95815=CARTESIAN_POINT('Origin',(8.52833113701624,-25.6742356128,7.18862868760432));
#95816=CARTESIAN_POINT('',(8.74359670241,-32.4742356128,7.39758828372));
#95817=CARTESIAN_POINT('Origin',(8.52833752869,-32.4742356128,7.18863018236));
#95818=CARTESIAN_POINT('',(8.74359670241,-28.8242356128,7.39758828372));
#95819=CARTESIAN_POINT('Origin',(-0.0657457778947,-28.8242356128,-1.15388688513));
#95820=CARTESIAN_POINT('',(0.0451717833072,-25.6742356128,11.1229180654));
#95821=CARTESIAN_POINT('Origin',(-0.0657457778946,-25.6742356128,-1.15388688513));
#95822=CARTESIAN_POINT('',(0.0451717833072,-32.4742356128,11.1229180654));
#95823=CARTESIAN_POINT('Origin',(-0.0657457778947,-32.4742356128,-1.15388688513));
#95824=CARTESIAN_POINT('',(0.0451717833071,-28.8242356128,11.1229180654));
#95825=CARTESIAN_POINT('Origin',(-15.6588697715,-25.6742356128,14.965390674));
#95826=CARTESIAN_POINT('',(8.30073298506,-25.1742356128,7.13507985462));
#95827=CARTESIAN_POINT('Ctrl Pts',(8.81393818057,-25.6742356128,7.09680280277));
#95828=CARTESIAN_POINT('Ctrl Pts',(8.81409597531014,-25.6430987071103,7.09679428198758));
#95829=CARTESIAN_POINT('Ctrl Pts',(8.81109093290262,-25.6115059429941,7.09701288121902));
#95830=CARTESIAN_POINT('Ctrl Pts',(8.80487037092342,-25.5800824415237,7.09746532919756));
#95831=CARTESIAN_POINT('Ctrl Pts',(8.79926072489547,-25.5517450146485,7.09787334265587));
#95832=CARTESIAN_POINT('Ctrl Pts',(8.79103561354454,-25.5235452886408,7.09847156569394));
#95833=CARTESIAN_POINT('Ctrl Pts',(8.78018861926916,-25.4959592212314,7.09926271867066));
#95834=CARTESIAN_POINT('Ctrl Pts',(8.77037287022121,-25.4709958158829,7.09997865516707));
#95835=CARTESIAN_POINT('Ctrl Pts',(8.75840870206946,-25.4465334581682,7.10085268219171));
#95836=CARTESIAN_POINT('Ctrl Pts',(8.74432821981368,-25.4229440144713,7.10188423921424));
#95837=CARTESIAN_POINT('Ctrl Pts',(8.73123668297153,-25.4010113799469,7.10284334462838));
#95838=CARTESIAN_POINT('Ctrl Pts',(8.71631480657571,-25.3798332969455,7.10393869376322));
#95839=CARTESIAN_POINT('Ctrl Pts',(8.69963101268627,-25.359720545253,7.10516680982952));
#95840=CARTESIAN_POINT('Ctrl Pts',(8.69317933739034,-25.3519428812463,7.10564172615479));
#95841=CARTESIAN_POINT('Ctrl Pts',(8.68646461977483,-25.3443245121491,7.10613646555696));
#95842=CARTESIAN_POINT('Ctrl Pts',(8.67949292808951,-25.3368836314267,7.10665067565743));
#95843=CARTESIAN_POINT('Ctrl Pts',(8.67647070290223,-25.3336580130044,7.10687358550303));
#95844=CARTESIAN_POINT('Ctrl Pts',(8.67316612602285,-25.3302224683051,7.10711784043832));
#95845=CARTESIAN_POINT('Ctrl Pts',(8.66993041923766,-25.3269524229621,7.10735706822193));
#95846=CARTESIAN_POINT('Ctrl Pts',(8.66677232332068,-25.3237608121235,7.10759055794669));
#95847=CARTESIAN_POINT('Ctrl Pts',(8.66368055276476,-25.3207264237881,7.1078192059096));
#95848=CARTESIAN_POINT('Ctrl Pts',(8.66101580561167,-25.3181635759878,7.10801593081068));
#95849=CARTESIAN_POINT('Ctrl Pts',(8.64724802689458,-25.3049222741409,7.10903233677742));
#95850=CARTESIAN_POINT('Ctrl Pts',(8.63225657618394,-25.2920046393027,7.11014168728378));
#95851=CARTESIAN_POINT('Ctrl Pts',(8.61600070173619,-25.2796661628299,7.11134761798622));
#95852=CARTESIAN_POINT('Ctrl Pts',(8.60677675522023,-25.2726650354873,7.11203189002197));
#95853=CARTESIAN_POINT('Ctrl Pts',(8.59714641349781,-25.2658508967218,7.11274721153374));
#95854=CARTESIAN_POINT('Ctrl Pts',(8.58710884486889,-25.259274077119,7.11349381184021));
#95855=CARTESIAN_POINT('Ctrl Pts',(8.5698814614288,-25.2479863442725,7.11477519483558));
#95856=CARTESIAN_POINT('Ctrl Pts',(8.55145176627244,-25.2373969109191,7.11614891068513));
#95857=CARTESIAN_POINT('Ctrl Pts',(8.53185116100626,-25.2277728047567,7.11761393892338));
#95858=CARTESIAN_POINT('Ctrl Pts',(8.52384812727395,-25.2238432298677,7.11821211792093));
#95859=CARTESIAN_POINT('Ctrl Pts',(8.51565041966796,-25.2200747426444,7.11882548312532));
#95860=CARTESIAN_POINT('Ctrl Pts',(8.50726250968196,-25.2164861229366,7.11945380371546));
#95861=CARTESIAN_POINT('Ctrl Pts',(8.50488129707811,-25.2154673630199,7.11963217531351));
#95862=CARTESIAN_POINT('Ctrl Pts',(8.50197597208091,-25.2142508838615,7.11984987911369));
#95863=CARTESIAN_POINT('Ctrl Pts',(8.49942431172375,-25.2132081626979,7.1200411607002));
#95864=CARTESIAN_POINT('Ctrl Pts',(8.49754711050464,-25.2124410553381,7.12018188241748));
#95865=CARTESIAN_POINT('Ctrl Pts',(8.49586208380619,-25.2117662483067,7.12030824103353));
#95866=CARTESIAN_POINT('Ctrl Pts',(8.49472562376124,-25.2113146890593,7.12039348309374));
#95867=CARTESIAN_POINT('Ctrl Pts',(8.48470395294944,-25.2073326941365,7.12114517504327));
#95868=CARTESIAN_POINT('Ctrl Pts',(8.47355138450343,-25.2032580976879,7.12198258088398));
#95869=CARTESIAN_POINT('Ctrl Pts',(8.4612079575769,-25.1993036718151,7.12291109578253));
#95870=CARTESIAN_POINT('Ctrl Pts',(8.44960457064268,-25.1955863302876,7.12378394233529));
#95871=CARTESIAN_POINT('Ctrl Pts',(8.43694804343264,-25.1919755178591,7.12473735944721));
#95872=CARTESIAN_POINT('Ctrl Pts',(8.42320929947104,-25.1886882300447,7.12577452498151));
#95873=CARTESIAN_POINT('Ctrl Pts',(8.41004691756789,-25.185538849158,7.12676817977974));
#95874=CARTESIAN_POINT('Ctrl Pts',(8.39589040114202,-25.182686711434,7.12783876345823));
#95875=CARTESIAN_POINT('Ctrl Pts',(8.38074527934273,-25.1803564605959,7.1289869922473));
#95876=CARTESIAN_POINT('Ctrl Pts',(8.36665346776027,-25.1781882736254,7.13005536422632));
#95877=CARTESIAN_POINT('Ctrl Pts',(8.35170527003246,-25.1764723672986,7.1311909953895));
#95878=CARTESIAN_POINT('Ctrl Pts',(8.33594155628545,-25.1754140609642,7.1323919600745));
#95879=CARTESIAN_POINT('Ctrl Pts',(8.32461548857318,-25.1746536786458,7.13325484096417));
#95880=CARTESIAN_POINT('Ctrl Pts',(8.3128690940841,-25.1742332866394,7.13415140342761));
#95881=CARTESIAN_POINT('Ctrl Pts',(8.30073298506,-25.1742356128,7.13507985462));
#95882=CARTESIAN_POINT('',(3.40300521133,-25.1742356128,-1.52767616996));
#95883=CARTESIAN_POINT('Origin',(-15.6588697715,-25.1742356128,14.965390674));
#95884=CARTESIAN_POINT('Origin',(3.40300521133,-25.6742356128,-1.52767616996));
#95885=CARTESIAN_POINT('Ctrl Pts',(8.30073298506,-25.1742356128,7.13507985462));
#95886=CARTESIAN_POINT('Ctrl Pts',(8.30073298506,-25.1742356128,7.13507985462));
#95887=CARTESIAN_POINT('Ctrl Pts',(8.30073298506,-25.1742356128,7.13507985462));
#95888=CARTESIAN_POINT('Ctrl Pts',(8.30073298506,-25.1742356128,7.13507985462));
#95889=CARTESIAN_POINT('Ctrl Pts',(8.30073298506,-25.1742356128,7.13507985462));
#95890=CARTESIAN_POINT('Ctrl Pts',(8.30073298506,-25.1742356128,7.13507985462));
#95891=CARTESIAN_POINT('Ctrl Pts',(8.4984544281,-25.174197715,7.11995353125));
#95892=CARTESIAN_POINT('Ctrl Pts',(8.49276880815,-25.1768387338,7.14348907236));
#95893=CARTESIAN_POINT('Ctrl Pts',(8.48739621864,-25.1782703109,7.1669182153));
#95894=CARTESIAN_POINT('Ctrl Pts',(8.48185217011,-25.1782703109,7.1903276789));
#95895=CARTESIAN_POINT('Ctrl Pts',(8.47614313121,-25.1768387338,7.21368444167));
#95896=CARTESIAN_POINT('Ctrl Pts',(8.47066320143,-25.174197715,7.23727979168));
#95897=CARTESIAN_POINT('Ctrl Pts',(8.70134899424,-25.2739717972,7.10492272115));
#95898=CARTESIAN_POINT('Ctrl Pts',(8.68923886464,-25.2513427762,7.15177407669));
#95899=CARTESIAN_POINT('Ctrl Pts',(8.6767502882,-25.2399151794,7.19877329204));
#95900=CARTESIAN_POINT('Ctrl Pts',(8.66568269835,-25.2399151794,7.24586328974));
#95901=CARTESIAN_POINT('Ctrl Pts',(8.65593998646,-25.2513427762,7.29347796257));
#95902=CARTESIAN_POINT('Ctrl Pts',(8.64594321094,-25.2739717972,7.34077222156));
#95903=CARTESIAN_POINT('Ctrl Pts',(8.81494578451,-25.4754097912,7.09674839301));
#95904=CARTESIAN_POINT('Ctrl Pts',(8.83671968197,-25.4572913208,7.15869208185));
#95905=CARTESIAN_POINT('Ctrl Pts',(8.84072845773,-25.4471049231,7.22634784813));
#95906=CARTESIAN_POINT('Ctrl Pts',(8.82507001711,-25.4471049231,7.29331987756));
#95907=CARTESIAN_POINT('Ctrl Pts',(8.79148126327,-25.4572913208,7.35218191877));
#95908=CARTESIAN_POINT('Ctrl Pts',(8.74450298325,-25.4754097912,7.39804592883));
#95909=CARTESIAN_POINT('Ctrl Pts',(8.81393818057,-25.6742356128,7.09680280277));
#95910=CARTESIAN_POINT('Ctrl Pts',(8.83380283672,-25.6742356128,7.15858566939));
#95911=CARTESIAN_POINT('Ctrl Pts',(8.83696093696,-25.6742356128,7.22574008976));
#95912=CARTESIAN_POINT('Ctrl Pts',(8.82141102617,-25.6742356128,7.29223268441));
#95913=CARTESIAN_POINT('Ctrl Pts',(8.78879978729,-25.6742356128,7.35102211263));
#95914=CARTESIAN_POINT('Ctrl Pts',(8.74359670241,-25.6742356128,7.39758828372));
#95915=CARTESIAN_POINT('Ctrl Pts',(8.74359670241,-25.6742356128,7.39758828372));
#95916=CARTESIAN_POINT('Ctrl Pts',(8.74372026636865,-25.6475507397519,7.39764771721947));
#95917=CARTESIAN_POINT('Ctrl Pts',(8.74182618313521,-25.6208162503538,7.39653602596286));
#95918=CARTESIAN_POINT('Ctrl Pts',(8.73801919658173,-25.5944358816126,7.39430757850375));
#95919=CARTESIAN_POINT('Ctrl Pts',(8.73421219462006,-25.5680554061009,7.39207912202535));
#95920=CARTESIAN_POINT('Ctrl Pts',(8.72849227567299,-25.5420290554374,7.38873390121572));
#95921=CARTESIAN_POINT('Ctrl Pts',(8.72098866821749,-25.5167170035454,7.38434111159174));
#95922=CARTESIAN_POINT('Ctrl Pts',(8.71348504486413,-25.4914048980248,7.37994831266077));
#95923=CARTESIAN_POINT('Ctrl Pts',(8.70419772727086,-25.466807095613,7.37450794139217));
#95924=CARTESIAN_POINT('Ctrl Pts',(8.69328040076856,-25.4432401846987,7.36810400637077));
#95925=CARTESIAN_POINT('Ctrl Pts',(8.68236303758426,-25.4196731946,7.36170004983228));
#95926=CARTESIAN_POINT('Ctrl Pts',(8.66981565635879,-25.3971371042455,7.35433252397831));
#95927=CARTESIAN_POINT('Ctrl Pts',(8.65581637278916,-25.3759048974086,7.34610023724638));
#95928=CARTESIAN_POINT('Ctrl Pts',(8.64227591227988,-25.3553685709052,7.33813776167824));
#95929=CARTESIAN_POINT('Ctrl Pts',(8.6273772855856,-25.3360518414704,7.32936635610616));
#95930=CARTESIAN_POINT('Ctrl Pts',(8.6113033813004,-25.3181628924002,7.31988858811994));
#95931=CARTESIAN_POINT('Ctrl Pts',(8.59486613553566,-25.2998695737937,7.3101965805699));
#95932=CARTESIAN_POINT('Ctrl Pts',(8.57720378186642,-25.2830667777551,7.29975760222087));
#95933=CARTESIAN_POINT('Ctrl Pts',(8.55853027393535,-25.2679387521626,7.28870277438831));
#95934=CARTESIAN_POINT('Ctrl Pts',(8.53975404846916,-25.2527275117021,7.27758713716363));
#95935=CARTESIAN_POINT('Ctrl Pts',(8.5199555841994,-25.2392096737772,7.26584898160584));
#95936=CARTESIAN_POINT('Ctrl Pts',(8.49937968702385,-25.2275283404032,7.25363349339433));
#95937=CARTESIAN_POINT('Ctrl Pts',(8.47873372599749,-25.2158072304309,7.24137640971136));
#95938=CARTESIAN_POINT('Ctrl Pts',(8.45730513048159,-25.2059351634624,7.22863884304467));
#95939=CARTESIAN_POINT('Ctrl Pts',(8.4353672412806,-25.1980110304246,7.21557761615551));
#95940=CARTESIAN_POINT('Ctrl Pts',(8.41288483366739,-25.1898902131798,7.20219219770616));
#95941=CARTESIAN_POINT('Ctrl Pts',(8.38986748854582,-25.1838151952435,7.18846686114024));
#95942=CARTESIAN_POINT('Ctrl Pts',(8.36663630941895,-25.179844349708,7.17458014983943));
#95943=CARTESIAN_POINT('Ctrl Pts',(8.34476122003766,-25.1761052970954,7.16150405717714));
#95944=CARTESIAN_POINT('Ctrl Pts',(8.3226966840604,-25.1742311488963,7.14828490547556));
#95945=CARTESIAN_POINT('Ctrl Pts',(8.30073298506,-25.1742356128,7.13507985462));
#95946=CARTESIAN_POINT('Origin',(-0.0657457778946,-25.6742356128,-1.15388688513));
#95947=CARTESIAN_POINT('',(0.0406546049764,-25.1742356128,10.6229384707));
#95948=CARTESIAN_POINT('Origin',(0.0406546049764,-25.6742356128,10.6229384707));
#95949=CARTESIAN_POINT('Origin',(-0.0657457778947,-25.1742356128,-1.15388688513));
#95950=CARTESIAN_POINT('Origin',(-1.33907057367E-16,-25.1742356128,0.729452270839));
#95951=CARTESIAN_POINT('',(-8.30073298506,-25.1742356128,7.13507985462));
#95952=CARTESIAN_POINT('',(-3.40300521133,-25.1742356128,-1.52767616996));
#95953=CARTESIAN_POINT('Origin',(15.6588697715,-25.1742356128,14.965390674));
#95954=CARTESIAN_POINT('Origin',(2.80638175951E-15,-25.1742356128,1.41673472726));
#95955=CARTESIAN_POINT('',(-0.0406546049764,-25.1742356128,10.6229384707));
#95956=CARTESIAN_POINT('Origin',(-5.68076154778E-15,-25.1742356128,6.12312211857));
#95957=CARTESIAN_POINT('Origin',(0.0657457778947,-25.1742356128,-1.15388688513));
#95958=CARTESIAN_POINT('Origin',(2.74514941955E-15,-25.6742356128,1.41673472726));
#95959=CARTESIAN_POINT('',(-3.78111690148,-25.6742356128,-1.85483293631));
#95960=CARTESIAN_POINT('Origin',(4.0774170491E-15,-25.6742356128,1.41673472726));
#95961=CARTESIAN_POINT('Origin',(-3.40300521133,-25.6742356128,-1.52767616996));
#95962=CARTESIAN_POINT('Origin',(3.69165330737E-15,-28.8242356128,1.41673472726));
#95963=CARTESIAN_POINT('',(-3.78111690148,-32.4742356128,-1.85483293631));
#95964=CARTESIAN_POINT('',(-3.78111690148,-28.8242356128,-1.85483293631));
#95965=CARTESIAN_POINT('Origin',(3.24465722568E-15,-32.4742356128,1.41673472726));
#95966=CARTESIAN_POINT('Origin',(15.6588697715,-25.6742356128,14.965390674));
#95967=CARTESIAN_POINT('',(-8.81393818057,-25.6742356128,7.09680280277));
#95968=CARTESIAN_POINT('Ctrl Pts',(-8.81393818057,-25.6742356128,7.09680280277));
#95969=CARTESIAN_POINT('Ctrl Pts',(-8.81494581646,-25.4754098599,7.09674839068));
#95970=CARTESIAN_POINT('Ctrl Pts',(-8.70134895175,-25.2739717119,7.10492272423));
#95971=CARTESIAN_POINT('Ctrl Pts',(-8.49845441271,-25.1741977344,7.11995353245));
#95972=CARTESIAN_POINT('Ctrl Pts',(-8.30073298506,-25.1742356128,7.13507985462));
#95973=CARTESIAN_POINT('Origin',(15.6588697715,-25.6742356128,14.965390674));
#95974=CARTESIAN_POINT('Origin',(15.6588697715,-28.8242356128,14.965390674));
#95975=CARTESIAN_POINT('',(-8.81393818057,-32.4742356128,7.09680280277));
#95976=CARTESIAN_POINT('',(-8.81393818057,-28.8242356128,7.09680280277));
#95977=CARTESIAN_POINT('Origin',(15.6588697715,-32.4742356128,14.965390674));
#95978=CARTESIAN_POINT('Origin',(-5.74199388774E-15,-25.6742356128,6.12312211857));
#95979=CARTESIAN_POINT('',(-0.0451717833072,-25.6742356128,11.1229180654));
#95980=CARTESIAN_POINT('Origin',(-5.76281056945E-15,-25.6742356128,6.12312211857));
#95981=CARTESIAN_POINT('Origin',(-0.0406546049764,-25.6742356128,10.6229384707));
#95982=CARTESIAN_POINT('Origin',(-6.14857431118E-15,-28.8242356128,6.12312211857));
#95983=CARTESIAN_POINT('',(-0.0451717833072,-32.4742356128,11.1229180654));
#95984=CARTESIAN_POINT('Origin',(-6.59557039287E-15,-32.4742356128,6.12312211857));
#95985=CARTESIAN_POINT('',(-0.0451717833072,-28.8242356128,11.1229180654));
#95986=CARTESIAN_POINT('Origin',(-8.52833752869,-28.8242356128,7.18863018236));
#95987=CARTESIAN_POINT('',(-8.74359670241,-25.6742356128,7.39758828372));
#95988=CARTESIAN_POINT('Origin',(-8.52833113701624,-25.6742356128,7.18862868760432));
#95989=CARTESIAN_POINT('',(-8.74359670241,-32.4742356128,7.39758828372));
#95990=CARTESIAN_POINT('',(-8.74359670241,-28.8242356128,7.39758828372));
#95991=CARTESIAN_POINT('Origin',(-8.52833752869,-32.4742356128,7.18863018236));
#95992=CARTESIAN_POINT('Origin',(0.0657457778947,-25.6742356128,-1.15388688513));
#95993=CARTESIAN_POINT('Ctrl Pts',(-8.74359670241,-25.6742356128,7.39758828372));
#95994=CARTESIAN_POINT('Ctrl Pts',(-8.74374103998485,-25.6425708684088,
7.39766117029625));
#95995=CARTESIAN_POINT('Ctrl Pts',(-8.74104638015217,-25.6104477310781,
7.39608617488609));
#95996=CARTESIAN_POINT('Ctrl Pts',(-8.7354771414879,-25.5785226691775,7.39283088384102));
#95997=CARTESIAN_POINT('Ctrl Pts',(-8.73040906011818,-25.5494704375891,
7.38986852562778));
#95998=CARTESIAN_POINT('Ctrl Pts',(-8.72295992326411,-25.5205822157641,
7.38551435667961));
#95999=CARTESIAN_POINT('Ctrl Pts',(-8.71313383437791,-25.4923697627127,
7.37976148770456));
#96000=CARTESIAN_POINT('Ctrl Pts',(-8.70468153488379,-25.4681017039341,
7.37481292962711));
#96001=CARTESIAN_POINT('Ctrl Pts',(-8.69446951826318,-25.4443321822236,
7.36882887446864));
#96002=CARTESIAN_POINT('Ctrl Pts',(-8.68253023474047,-25.4214038181183,
7.3618220078867));
#96003=CARTESIAN_POINT('Ctrl Pts',(-8.67075128078371,-25.3987833531141,
7.35490923471293));
#96004=CARTESIAN_POINT('Ctrl Pts',(-8.65728988089475,-25.3769813332839,
7.34700019558017));
#96005=CARTESIAN_POINT('Ctrl Pts',(-8.64221836816086,-25.3563387689072,
7.33813082388733));
#96006=CARTESIAN_POINT('Ctrl Pts',(-8.63738810977467,-25.3497230481463,
7.33528828526789));
#96007=CARTESIAN_POINT('Ctrl Pts',(-8.63239278338873,-25.3432263804671,
7.33234727894179));
#96008=CARTESIAN_POINT('Ctrl Pts',(-8.62723614053898,-25.3368600324647,
7.32930928634434));
#96009=CARTESIAN_POINT('Ctrl Pts',(-8.62461032881768,-25.333618227342,7.32776231153843));
#96010=CARTESIAN_POINT('Ctrl Pts',(-8.62174269443592,-25.3301699453249,
7.32607232011319));
#96011=CARTESIAN_POINT('Ctrl Pts',(-8.61893519950626,-25.3268883248504,
7.32441745480467));
#96012=CARTESIAN_POINT('Ctrl Pts',(-8.61622925699588,-25.3237254068158,
7.32282244911472));
#96013=CARTESIAN_POINT('Ctrl Pts',(-8.61357983367571,-25.3207168303973,
7.32126046002638));
#96014=CARTESIAN_POINT('Ctrl Pts',(-8.61128536912057,-25.3181634673016,
7.31990782820919));
#96015=CARTESIAN_POINT('Ctrl Pts',(-8.59929941137436,-25.3048250602617,
7.31284187124298));
#96016=CARTESIAN_POINT('Ctrl Pts',(-8.58625654488145,-25.2918288567523,
7.3051443219223));
#96017=CARTESIAN_POINT('Ctrl Pts',(-8.57212647692136,-25.2794305292251,
7.29679382196662));
#96018=CARTESIAN_POINT('Ctrl Pts',(-8.56421120807483,-25.2724853329314,
7.2921161054589));
#96019=CARTESIAN_POINT('Ctrl Pts',(-8.55595540779658,-25.2657282394864,
7.28723384786007));
#96020=CARTESIAN_POINT('Ctrl Pts',(-8.54735934678809,-25.259207553683,7.28214644639095));
#96021=CARTESIAN_POINT('Ctrl Pts',(-8.53238762194693,-25.2478505014786,
7.27328573973973));
#96022=CARTESIAN_POINT('Ctrl Pts',(-8.51638126776519,-25.2372098719035,
7.26380132803334));
#96023=CARTESIAN_POINT('Ctrl Pts',(-8.4993730392377,-25.2275526372549,7.25370744627357));
#96024=CARTESIAN_POINT('Ctrl Pts',(-8.49258297210632,-25.2236972521123,
7.2496777417894));
#96025=CARTESIAN_POINT('Ctrl Pts',(-8.4856336790979,-25.2199987375441,7.24555115737597));
#96026=CARTESIAN_POINT('Ctrl Pts',(-8.4785291407219,-25.2164745981546,7.24132967662755));
#96027=CARTESIAN_POINT('Ctrl Pts',(-8.47646322137075,-25.215449818306,7.24010211780429));
#96028=CARTESIAN_POINT('Ctrl Pts',(-8.47395268214777,-25.2142311697352,
7.23861008609302));
#96029=CARTESIAN_POINT('Ctrl Pts',(-8.47174800998708,-25.2131866536585,
7.23729953917551));
#96030=CARTESIAN_POINT('Ctrl Pts',(-8.47015655922779,-25.2124326658626,
7.2363535160324));
#96031=CARTESIAN_POINT('Ctrl Pts',(-8.46872511422753,-25.2117677253727,
7.2355024531919));
#96032=CARTESIAN_POINT('Ctrl Pts',(-8.46774142009499,-25.2113143951645,
7.23491753911709));
#96033=CARTESIAN_POINT('Ctrl Pts',(-8.45887145042537,-25.2072267168266,
7.22964336909694));
#96034=CARTESIAN_POINT('Ctrl Pts',(-8.44903341435114,-25.2030683007582,
7.22378969990896));
#96035=CARTESIAN_POINT('Ctrl Pts',(-8.43817822310785,-25.1990544953082,
7.21732358184192));
#96036=CARTESIAN_POINT('Ctrl Pts',(-8.42798831593375,-25.1952866846789,
7.21125375392244));
#96037=CARTESIAN_POINT('Ctrl Pts',(-8.41690143527307,-25.1916466537825,
7.20464384498518));
#96038=CARTESIAN_POINT('Ctrl Pts',(-8.40489619864105,-25.188352056581,7.19747738556042));
#96039=CARTESIAN_POINT('Ctrl Pts',(-8.3933971585147,-25.1851963748913,7.19061309733228));
#96040=CARTESIAN_POINT('Ctrl Pts',(-8.38105487920422,-25.1823579194766,
7.18323779100804));
#96041=CARTESIAN_POINT('Ctrl Pts',(-8.36787853944442,-25.1800609103949,
7.17535300675156));
#96042=CARTESIAN_POINT('Ctrl Pts',(-8.35560155307287,-25.1779206840722,
7.16800639983157));
#96043=CARTESIAN_POINT('Ctrl Pts',(-8.34260004343601,-25.1762509850684,
7.16021723063684));
#96044=CARTESIAN_POINT('Ctrl Pts',(-8.32891385869611,-25.1752566994474,
7.15200547873626));
#96045=CARTESIAN_POINT('Ctrl Pts',(-8.31981484133295,-25.174595666274,7.14654604102258));
#96046=CARTESIAN_POINT('Ctrl Pts',(-8.3104138424029,-25.1742336464764,7.14090019430669));
#96047=CARTESIAN_POINT('Ctrl Pts',(-8.30073298506,-25.1742356128,7.13507985462));
#96048=CARTESIAN_POINT('Origin',(0.0657457778947,-25.6742356128,-1.15388688513));
#96049=CARTESIAN_POINT('Ctrl Pts',(-8.30073298506,-25.1742356128,7.13507985462));
#96050=CARTESIAN_POINT('Ctrl Pts',(-8.30073298506,-25.1742356128,7.13507985462));
#96051=CARTESIAN_POINT('Ctrl Pts',(-8.30073298506,-25.1742356128,7.13507985462));
#96052=CARTESIAN_POINT('Ctrl Pts',(-8.30073298506,-25.1742356128,7.13507985462));
#96053=CARTESIAN_POINT('Ctrl Pts',(-8.30073298506,-25.1742356128,7.13507985462));
#96054=CARTESIAN_POINT('Ctrl Pts',(-8.30073298506,-25.1742356128,7.13507985462));
#96055=CARTESIAN_POINT('Ctrl Pts',(-8.47066318824,-25.1741977344,7.23727978366));
#96056=CARTESIAN_POINT('Ctrl Pts',(-8.47614311863,-25.1768387543,7.2136844367));
#96057=CARTESIAN_POINT('Ctrl Pts',(-8.48185215775,-25.1782703319,7.19032767617));
#96058=CARTESIAN_POINT('Ctrl Pts',(-8.48739620589,-25.1782703319,7.16691821418));
#96059=CARTESIAN_POINT('Ctrl Pts',(-8.49276879436,-25.1768387543,7.14348907246));
#96060=CARTESIAN_POINT('Ctrl Pts',(-8.49845441271,-25.1741977344,7.11995353245));
#96061=CARTESIAN_POINT('Ctrl Pts',(-8.64594317412,-25.2739717119,7.34077220006));
#96062=CARTESIAN_POINT('Ctrl Pts',(-8.65593994326,-25.2513426907,7.29347794093));
#96063=CARTESIAN_POINT('Ctrl Pts',(-8.66568265086,-25.2399150938,7.2458632715));
#96064=CARTESIAN_POINT('Ctrl Pts',(-8.67675023931,-25.2399150938,7.1987732799));
#96065=CARTESIAN_POINT('Ctrl Pts',(-8.68923881751,-25.2513426907,7.15177407204));
#96066=CARTESIAN_POINT('Ctrl Pts',(-8.70134895175,-25.2739717119,7.10492272423));
#96067=CARTESIAN_POINT('Ctrl Pts',(-8.74450301091,-25.4754098599,7.39804594503));
#96068=CARTESIAN_POINT('Ctrl Pts',(-8.79148129659,-25.4572913909,7.35218193136));
#96069=CARTESIAN_POINT('Ctrl Pts',(-8.82507005415,-25.4471049939,7.29331988562));
#96070=CARTESIAN_POINT('Ctrl Pts',(-8.84072849584,-25.4471049939,7.22634785159));
#96071=CARTESIAN_POINT('Ctrl Pts',(-8.83671971824,-25.4572913909,7.15869208165));
#96072=CARTESIAN_POINT('Ctrl Pts',(-8.81494581646,-25.4754098599,7.09674839068));
#96073=CARTESIAN_POINT('Ctrl Pts',(-8.74359670241,-25.6742356128,7.39758828372));
#96074=CARTESIAN_POINT('Ctrl Pts',(-8.78879978729,-25.6742356128,7.35102211263));
#96075=CARTESIAN_POINT('Ctrl Pts',(-8.82141102617,-25.6742356128,7.29223268441));
#96076=CARTESIAN_POINT('Ctrl Pts',(-8.83696093696,-25.6742356128,7.22574008976));
#96077=CARTESIAN_POINT('Ctrl Pts',(-8.83380283672,-25.6742356128,7.15858566939));
#96078=CARTESIAN_POINT('Ctrl Pts',(-8.81393818057,-25.6742356128,7.09680280277));
#96079=CARTESIAN_POINT('Origin',(0.0657457778947,-28.8242356128,-1.15388688513));
#96080=CARTESIAN_POINT('Origin',(0.0657457778947,-32.4742356128,-1.15388688513));
#96081=CARTESIAN_POINT('Origin',(-2.68618205273E-16,-26.2742356128,0.729452270839));
#96082=CARTESIAN_POINT('',(-7.90115867216,-26.2742356128,11.6700302451));
#96083=CARTESIAN_POINT('',(-9.22598000443009,-26.274235669025,12.8949853715999));
#96084=CARTESIAN_POINT('',(-9.09620098718,-26.2742356128,12.7749892117));
#96085=CARTESIAN_POINT('',(-11.4035900518,-26.2742356128,8.02142239733));
#96086=CARTESIAN_POINT('Origin',(-3.57591647086E-14,-26.2742356128,0.580061096522));
#96087=CARTESIAN_POINT('',(-12.6175523599,-26.2742356128,9.14387515104));
#96088=CARTESIAN_POINT('',(-12.1305681918,-26.2742356128,8.69360028097));
#96089=CARTESIAN_POINT('',(-12.1784262599,-26.2742356128,9.98548517727));
#96090=CARTESIAN_POINT('Origin',(-10.0415172382,-26.2742356128,8.33514586886));
#96091=CARTESIAN_POINT('Origin',(-2.00838475998E-15,-26.2742356128,0.580061096523));
#96092=CARTESIAN_POINT('Origin',(-12.1305681918,-25.9742356128,8.69360028097));
#96093=CARTESIAN_POINT('',(-12.6068339548724,-26.2541477093856,8.98696687274956));
#96094=CARTESIAN_POINT('',(-12.5655736216481,-25.9742356128984,8.68722821702829));
#96095=CARTESIAN_POINT('Ctrl Pts',(-12.6068339569,-26.2541477174,8.98696686913));
#96096=CARTESIAN_POINT('Ctrl Pts',(-12.602271199,-26.244718344,8.94944232356));
#96097=CARTESIAN_POINT('Ctrl Pts',(-12.5976340417,-26.2325138521,8.912882128));
#96098=CARTESIAN_POINT('Ctrl Pts',(-12.592997343,-26.2175047318,8.87772639907));
#96099=CARTESIAN_POINT('Ctrl Pts',(-12.5863327646,-26.191160811,8.82889624954));
#96100=CARTESIAN_POINT('Ctrl Pts',(-12.5802806769,-26.1586266769,8.78631135752));
#96101=CARTESIAN_POINT('Ctrl Pts',(-12.5784179469,-26.1475421121,8.77337100062));
#96102=CARTESIAN_POINT('Ctrl Pts',(-12.5749839513,-26.1246988195,8.74977888646));
#96103=CARTESIAN_POINT('Ctrl Pts',(-12.5720318185,-26.0996123734,8.72988564417));
#96104=CARTESIAN_POINT('Ctrl Pts',(-12.5707272399,-26.0868775377,8.72117067463));
#96105=CARTESIAN_POINT('Ctrl Pts',(-12.568480527,-26.061055694,8.7062606411));
#96106=CARTESIAN_POINT('Ctrl Pts',(-12.566907631,-26.033788263,8.69593652529));
#96107=CARTESIAN_POINT('Ctrl Pts',(-12.5663159136,-26.020173083,8.69206958938));
#96108=CARTESIAN_POINT('Ctrl Pts',(-12.5658096281,-26.0027489841,8.68876644826));
#96109=CARTESIAN_POINT('Ctrl Pts',(-12.5656142634,-25.9851944876,8.68749304576));
#96110=CARTESIAN_POINT('Ctrl Pts',(-12.5655871714,-25.981542709,8.68731649095));
#96111=CARTESIAN_POINT('Ctrl Pts',(-12.5655736257,-25.9778891268,8.68722821403));
#96112=CARTESIAN_POINT('Ctrl Pts',(-12.5655736197,-25.9742356128,8.68722821523));
#96113=CARTESIAN_POINT('Ctrl Pts',(-12.6175523599,-26.2742356128,9.14387515104));
#96114=CARTESIAN_POINT('Ctrl Pts',(-12.6172775701366,-26.2742356128,9.1204109896849));
#96115=CARTESIAN_POINT('Ctrl Pts',(-12.6163614798089,-26.2727853712571,
9.09667519636503));
#96116=CARTESIAN_POINT('Ctrl Pts',(-12.6148425376273,-26.2699936097463,
9.07290148779792));
#96117=CARTESIAN_POINT('Ctrl Pts',(-12.6143935062009,-26.2691683060127,
9.06587347685785));
#96118=CARTESIAN_POINT('Ctrl Pts',(-12.6138920543085,-26.2682256034708,
9.05884197806186));
#96119=CARTESIAN_POINT('Ctrl Pts',(-12.6133398078109,-26.2671678572136,
9.05181269741915));
#96120=CARTESIAN_POINT('Ctrl Pts',(-12.6116358448962,-26.2639041689815,
9.03012377121524));
#96121=CARTESIAN_POINT('Ctrl Pts',(-12.6094465737123,-26.2595469161348,
9.00845340393981));
#96122=CARTESIAN_POINT('Ctrl Pts',(-12.6068339507173,-26.2541476931765,
8.9869668790268));
#96123=CARTESIAN_POINT('',(-11.607257429,-25.9742356128,7.80115074806));
#96124=CARTESIAN_POINT('Origin',(-11.4035900518,-25.9742356128,8.02142239733));
#96125=CARTESIAN_POINT('',(-12.3599175224,-25.9742356128,8.49707465678));
#96126=CARTESIAN_POINT('Origin',(-13.1616800929,-23.1742356128,9.23839965433));
#96127=CARTESIAN_POINT('',(-12.5655736249,-23.4742356128,8.68722822002));
#96128=CARTESIAN_POINT('',(-11.607257429,-23.4742356128,7.80115074806));
#96129=CARTESIAN_POINT('',(-3.17376422771,-23.4742356128,0.00338173602688));
#96130=CARTESIAN_POINT('',(-12.5655736249,-27.9742356128,8.68722822002));
#96131=CARTESIAN_POINT('',(-11.607257429,-24.7242356128,7.80115074806));
#96132=CARTESIAN_POINT('Origin',(-3.57224253046E-14,-25.9742356128,0.580061096522));
#96133=CARTESIAN_POINT('',(-7.72708272879,-25.9742356128,11.4256993917));
#96134=CARTESIAN_POINT('Origin',(-7.90115867216,-25.9742356128,11.6700302451));
#96135=CARTESIAN_POINT('',(-11.1523495973,-25.9742356128,7.85747657088));
#96136=CARTESIAN_POINT('Origin',(-3.39552160364E-14,-25.9742356128,0.580061096522));
#96137=CARTESIAN_POINT('Origin',(-11.4035900518,-25.9742356128,8.02142239733));
#96138=CARTESIAN_POINT('Origin',(-11.4035900518,-25.9742356128,8.02142239733));
#96139=CARTESIAN_POINT('Origin',(-11.4035900518,-25.9742356128,8.02142239733));
#96140=CARTESIAN_POINT('Origin',(-11.4035900518,-24.7242356128,8.02142239733));
#96141=CARTESIAN_POINT('',(-11.1523495973,-23.4742356128,7.85747657088));
#96142=CARTESIAN_POINT('Origin',(-11.4035900518,-23.4742356128,8.02142239733));
#96143=CARTESIAN_POINT('',(-11.1523495973,-24.7267356128,7.85747657088));
#96144=CARTESIAN_POINT('Origin',(-3.37715190165E-14,-24.4742356128,0.580061096522));
#96145=CARTESIAN_POINT('',(-7.72708272879,-23.4742356128,11.4256993917));
#96146=CARTESIAN_POINT('',(-7.72708272879,-24.7242356128,11.4256993917));
#96147=CARTESIAN_POINT('Origin',(-3.36399067654E-14,-23.4742356128,0.580061096522));
#96148=CARTESIAN_POINT('Origin',(-9.09620098718,-25.9742356128,12.7749892117));
#96149=CARTESIAN_POINT('',(-8.93233349645,-25.9742356128,13.0320605967));
#96150=CARTESIAN_POINT('Ctrl Pts',(-8.93233349645,-25.9742356128,13.0320605967));
#96151=CARTESIAN_POINT('Ctrl Pts',(-8.93233349645,-25.9890568327864,13.0320605967));
#96152=CARTESIAN_POINT('Ctrl Pts',(-8.93344543935767,-26.0038788180243,
13.0315888128132));
#96153=CARTESIAN_POINT('Ctrl Pts',(-8.93564750676488,-26.018509087112,13.0306516936333));
#96154=CARTESIAN_POINT('Ctrl Pts',(-8.93798761514531,-26.034056483703,13.0296558292747));
#96155=CARTESIAN_POINT('Ctrl Pts',(-8.94155846689529,-26.0493869490561,
13.0281345264418));
#96156=CARTESIAN_POINT('Ctrl Pts',(-8.94628177617279,-26.0642939979475,
13.0261107034094));
#96157=CARTESIAN_POINT('Ctrl Pts',(-8.95118424470664,-26.0797664842551,
13.0240101149975));
#96158=CARTESIAN_POINT('Ctrl Pts',(-8.9573276962761,-26.0947828330173,13.0213682483627));
#96159=CARTESIAN_POINT('Ctrl Pts',(-8.96457850957973,-26.1091429358216,
13.0182248593873));
#96160=CARTESIAN_POINT('Ctrl Pts',(-8.97222041741152,-26.1242775941682,
13.014911922228));
#96161=CARTESIAN_POINT('Ctrl Pts',(-8.98109059226912,-26.1386817706972,
13.0110424603843));
#96162=CARTESIAN_POINT('Ctrl Pts',(-8.99099940321383,-26.1521692986935,
13.0066739274749));
#96163=CARTESIAN_POINT('Ctrl Pts',(-8.99289007084896,-26.1547428095621,
13.0058403820747));
#96164=CARTESIAN_POINT('Ctrl Pts',(-8.99481848775625,-26.1572830840322,
13.0049886908228));
#96165=CARTESIAN_POINT('Ctrl Pts',(-8.9967832607327,-26.1597890245021,13.0041192827899));
#96166=CARTESIAN_POINT('Ctrl Pts',(-9.00694335034053,-26.1727475596766,
12.9996234638704));
#96167=CARTESIAN_POINT('Ctrl Pts',(-9.0180777154112,-26.1847862798302,12.9946527566583));
#96168=CARTESIAN_POINT('Ctrl Pts',(-9.02998776274932,-26.1957776113637,
12.9892701764838));
#96169=CARTESIAN_POINT('Ctrl Pts',(-9.03423770921764,-26.1996997259706,
12.9873494723124));
#96170=CARTESIAN_POINT('Ctrl Pts',(-9.03858641957574,-26.203488948385,12.9853763532502));
#96171=CARTESIAN_POINT('Ctrl Pts',(-9.04302503821336,-26.2071411042599,
12.9833537344883));
#96172=CARTESIAN_POINT('Ctrl Pts',(-9.05733192261861,-26.2189130036273,
12.9768342798594));
#96173=CARTESIAN_POINT('Ctrl Pts',(-9.07257322609965,-26.2292583824396,
12.9697996826004));
#96174=CARTESIAN_POINT('Ctrl Pts',(-9.08845512475273,-26.2380574138996,
12.9623517337336));
#96175=CARTESIAN_POINT('Ctrl Pts',(-9.10541279720069,-26.2474524551738,
12.9543992917712));
#96176=CARTESIAN_POINT('Ctrl Pts',(-9.12310069284028,-26.2550849446076,
12.9459753050102));
#96177=CARTESIAN_POINT('Ctrl Pts',(-9.14117969848556,-26.2608654055676,
12.9372106237479));
#96178=CARTESIAN_POINT('Ctrl Pts',(-9.1469184542949,-26.2627002771621,12.9344284814942));
#96179=CARTESIAN_POINT('Ctrl Pts',(-9.15269675618503,-26.2643489154705,
12.9316120798377));
#96180=CARTESIAN_POINT('Ctrl Pts',(-9.15850413396806,-26.2658094227087,
12.928765815912));
#96181=CARTESIAN_POINT('Ctrl Pts',(-9.17863028160214,-26.2708709815385,
12.9189017550375));
#96182=CARTESIAN_POINT('Ctrl Pts',(-9.19910546511503,-26.2736699194545,
12.9086770906661));
#96183=CARTESIAN_POINT('Ctrl Pts',(-9.21950805504983,-26.2741583270136,
12.8982876942716));
#96184=CARTESIAN_POINT('Ctrl Pts',(-9.22166632400898,-26.274209992752,12.8971886616579));
#96185=CARTESIAN_POINT('Ctrl Pts',(-9.22382380187443,-26.2742358404664,
12.8960878053211));
#96186=CARTESIAN_POINT('Ctrl Pts',(-9.22598000443021,-26.2742358377001,
12.8949853715998));
#96187=CARTESIAN_POINT('',(-7.69749129497,-25.9742356128,11.8903018944));
#96188=CARTESIAN_POINT('',(-8.68674913995,-25.9742356128,12.8049886066));
#96189=CARTESIAN_POINT('Origin',(-7.90115867216,-25.9742356128,11.6700302451));
#96190=CARTESIAN_POINT('Origin',(-7.90115867216,-25.9742356128,11.6700302451));
#96191=CARTESIAN_POINT('Origin',(-7.90115867216,-25.9742356128,11.6700302451));
#96192=CARTESIAN_POINT('Origin',(-7.90115867216,-24.7242356128,11.6700302451));
#96193=CARTESIAN_POINT('',(-7.69749129497,-23.4742356128,11.8903018944));
#96194=CARTESIAN_POINT('Origin',(-7.90115867216,-23.4742356128,11.6700302451));
#96195=CARTESIAN_POINT('',(-7.69749129497,-24.7267356128,11.8903018944));
#96196=CARTESIAN_POINT('Origin',(-9.64366495121,-23.1742356128,13.6897712562));
#96197=CARTESIAN_POINT('',(-8.93233349645,-23.4742356128,13.0320605967));
#96198=CARTESIAN_POINT('',(-8.93233349645,-27.9742356128,13.0320605967));
#96199=CARTESIAN_POINT('',(0.393995566301,-23.4742356128,4.40875848149));
#96200=CARTESIAN_POINT('Origin',(-2.68618205273E-16,-26.2742356128,0.729452270839));
#96201=CARTESIAN_POINT('',(11.4035900518,-26.2742356128,8.02142239733));
#96202=CARTESIAN_POINT('',(12.6175523516746,-26.27423561115,9.1438751395306));
#96203=CARTESIAN_POINT('',(12.1305681918,-26.2742356128,8.69360028097));
#96204=CARTESIAN_POINT('',(7.90115867216,-26.2742356128,11.6700302451));
#96205=CARTESIAN_POINT('Origin',(-4.37527704859E-14,-26.2742356128,0.580061096522));
#96206=CARTESIAN_POINT('',(9.22598003749396,-26.2742356128,12.8949854022109));
#96207=CARTESIAN_POINT('',(9.09620098718,-26.2742356128,12.7749892117));
#96208=CARTESIAN_POINT('',(12.1784262599,-26.2742356128,9.98548517727));
#96209=CARTESIAN_POINT('Origin',(1.54432891882E-15,-26.2742356128,0.580061096523));
#96210=CARTESIAN_POINT('Origin',(10.0415172382,-26.2742356128,8.33514586886));
#96211=CARTESIAN_POINT('Origin',(9.09620098718,-25.9742356128,12.7749892117));
#96212=CARTESIAN_POINT('',(8.93233349645,-25.9742356128,13.0320605967));
#96213=CARTESIAN_POINT('Ctrl Pts',(9.22598003749,-26.2742356128,12.8949854022));
#96214=CARTESIAN_POINT('Ctrl Pts',(9.18809325963,-26.2742357357,12.9143563956));
#96215=CARTESIAN_POINT('Ctrl Pts',(9.14988050464,-26.2675847856,12.9333199946));
#96216=CARTESIAN_POINT('Ctrl Pts',(9.112555303,-26.2543622577,12.9512548511));
#96217=CARTESIAN_POINT('Ctrl Pts',(9.03207275784,-26.2094852035,12.9888169711));
#96218=CARTESIAN_POINT('Ctrl Pts',(8.97065416936,-26.1347652578,13.0157974347));
#96219=CARTESIAN_POINT('Ctrl Pts',(8.9450884596,-26.0844303721,13.0266425468));
#96220=CARTESIAN_POINT('Ctrl Pts',(8.93233349646,-26.0293225561,13.0320605967));
#96221=CARTESIAN_POINT('Ctrl Pts',(8.93233349645,-25.9742356128,13.0320605967));
#96222=CARTESIAN_POINT('',(7.69749129497,-25.9742356128,11.8903018944));
#96223=CARTESIAN_POINT('Origin',(7.90115867216,-25.9742356128,11.6700302451));
#96224=CARTESIAN_POINT('',(8.68674913995,-25.9742356128,12.8049886066));
#96225=CARTESIAN_POINT('Origin',(9.64366495121,-23.1742356128,13.6897712562));
#96226=CARTESIAN_POINT('',(8.93233349645,-23.4742356128,13.0320605967));
#96227=CARTESIAN_POINT('',(7.69749129497,-23.4742356128,11.8903018944));
#96228=CARTESIAN_POINT('',(-0.408787176222,-23.4742356128,4.39508187623));
#96229=CARTESIAN_POINT('',(8.93233349645,-27.9742356128,13.0320605967));
#96230=CARTESIAN_POINT('',(7.69749129497,-24.7242356128,11.8903018944));
#96231=CARTESIAN_POINT('Origin',(7.90115867216,-25.9742356128,11.6700302451));
#96232=CARTESIAN_POINT('',(7.72708272879,-25.9742356128,11.4256993917));
#96233=CARTESIAN_POINT('Origin',(7.90115867216,-25.9742356128,11.6700302451));
#96234=CARTESIAN_POINT('Origin',(7.90115867216,-25.9742356128,11.6700302451));
#96235=CARTESIAN_POINT('Origin',(7.90115867216,-24.7242356128,11.6700302451));
#96236=CARTESIAN_POINT('Origin',(7.90115867216,-23.4742356128,11.6700302451));
#96237=CARTESIAN_POINT('',(7.72708272879,-24.7267356128,11.4256993917));
#96238=CARTESIAN_POINT('Origin',(-3.37715190165E-14,-24.4742356128,0.580061096522));
#96239=CARTESIAN_POINT('',(11.1523495973,-25.9742356128,7.85747657088));
#96240=CARTESIAN_POINT('Origin',(-4.37160310819E-14,-25.9742356128,0.580061096522));
#96241=CARTESIAN_POINT('',(11.1523495973,-24.7242356128,7.85747657088));
#96242=CARTESIAN_POINT('Origin',(-4.37160310819E-14,-25.9742356128,0.580061096522));
#96243=CARTESIAN_POINT('Origin',(11.4035900518,-25.9742356128,8.02142239733));
#96244=CARTESIAN_POINT('Origin',(12.1305681918,-25.9742356128,8.69360028097));
#96245=CARTESIAN_POINT('',(12.6068339233452,-26.2541477670181,8.98696693402157));
#96246=CARTESIAN_POINT('Ctrl Pts',(12.6068339453758,-26.254147742503,8.98696694713534));
#96247=CARTESIAN_POINT('Ctrl Pts',(12.609740724862,-26.2601548567899,9.01087250247576));
#96248=CARTESIAN_POINT('Ctrl Pts',(12.6121229018983,-26.2648728878816,9.03500586221848));
#96249=CARTESIAN_POINT('Ctrl Pts',(12.6138969346234,-26.2682287168868,9.05914080022458));
#96250=CARTESIAN_POINT('Ctrl Pts',(12.6144682432968,-26.2693094264984,9.06691320443121));
#96251=CARTESIAN_POINT('Ctrl Pts',(12.6149767251104,-26.2702485354808,9.07468576079593));
#96252=CARTESIAN_POINT('Ctrl Pts',(12.6154203387632,-26.27104275443,9.0824507415481));
#96253=CARTESIAN_POINT('Ctrl Pts',(12.6165958818517,-26.2731473754007,9.10302736131617));
#96254=CARTESIAN_POINT('Ctrl Pts',(12.6173143352754,-26.2742356003459,9.12355292911173));
#96255=CARTESIAN_POINT('Ctrl Pts',(12.6175523434,-26.2742356062,9.14387513582));
#96256=CARTESIAN_POINT('',(12.5655736249,-25.9742356128,8.68722822002));
#96257=CARTESIAN_POINT('Ctrl Pts',(12.5655736249,-25.9742356128,8.68722822002));
#96258=CARTESIAN_POINT('Ctrl Pts',(12.5655736249,-26.0013830382,8.68722822002));
#96259=CARTESIAN_POINT('Ctrl Pts',(12.566321511,-26.0285303094,8.69210196752));
#96260=CARTESIAN_POINT('Ctrl Pts',(12.5678174566,-26.0548464782,8.70184791871));
#96261=CARTESIAN_POINT('Ctrl Pts',(12.5710356589,-26.0928453409,8.7230882249));
#96262=CARTESIAN_POINT('Ctrl Pts',(12.5753569082,-26.1268141304,8.75236686589));
#96263=CARTESIAN_POINT('Ctrl Pts',(12.5769602275,-26.1380192113,8.76332897983));
#96264=CARTESIAN_POINT('Ctrl Pts',(12.5804314507,-26.1598522682,8.78731738945));
#96265=CARTESIAN_POINT('Ctrl Pts',(12.5842177446,-26.179372288,8.81410290281));
#96266=CARTESIAN_POINT('Ctrl Pts',(12.5862189463,-26.1887463534,8.82844547636));
#96267=CARTESIAN_POINT('Ctrl Pts',(12.5914446459,-26.2110918433,8.86644043173));
#96268=CARTESIAN_POINT('Ctrl Pts',(12.5968838275,-26.2294331381,8.90752664916));
#96269=CARTESIAN_POINT('Ctrl Pts',(12.6002199949,-26.2391192104,8.93339289159));
#96270=CARTESIAN_POINT('Ctrl Pts',(12.6035463933,-26.2473540241,8.95993044556));
#96271=CARTESIAN_POINT('Ctrl Pts',(12.6068338975,-26.2541477512,8.98696693379));
#96272=CARTESIAN_POINT('',(11.607257429,-25.9742356128,7.80115074806));
#96273=CARTESIAN_POINT('',(12.3599175224,-25.9742356128,8.49707465678));
#96274=CARTESIAN_POINT('Origin',(11.4035900518,-25.9742356128,8.02142239733));
#96275=CARTESIAN_POINT('Origin',(11.4035900518,-25.9742356128,8.02142239733));
#96276=CARTESIAN_POINT('Origin',(11.4035900518,-25.9742356128,8.02142239733));
#96277=CARTESIAN_POINT('Origin',(11.4035900518,-24.7242356128,8.02142239733));
#96278=CARTESIAN_POINT('',(11.607257429,-23.4742356128,7.80115074806));
#96279=CARTESIAN_POINT('Origin',(11.4035900518,-23.4742356128,8.02142239733));
#96280=CARTESIAN_POINT('',(11.607257429,-24.7267356128,7.80115074806));
#96281=CARTESIAN_POINT('Origin',(13.1616800929,-23.1742356128,9.23839965433));
#96282=CARTESIAN_POINT('',(12.5655736249,-23.4742356128,8.68722822002));
#96283=CARTESIAN_POINT('',(12.5655736249,-27.9742356128,8.68722822002));
#96284=CARTESIAN_POINT('',(3.26251388724,-23.4742356128,0.0854413675889));
#96285=CARTESIAN_POINT('Origin',(3.59394702409,-23.1742356128,-9.19678210318));
#96286=CARTESIAN_POINT('',(3.59394702409,-23.4742356128,-6.76017690617));
#96287=CARTESIAN_POINT('',(3.59394702409,-23.4742356128,-8.84845722572));
#96288=CARTESIAN_POINT('',(3.59394702409,-23.4742356128,3.49118372723));
#96289=CARTESIAN_POINT('',(3.59394702409,-25.9742356128,-8.84845722572));
#96290=CARTESIAN_POINT('',(3.59394702409,-27.9742356128,-8.84845722572));
#96291=CARTESIAN_POINT('',(3.59394702409,-25.9742356128,-6.76017690617));
#96292=CARTESIAN_POINT('',(3.59394702409,-25.9742356128,-8.53006468251));
#96293=CARTESIAN_POINT('',(3.59394702409,-24.7242356128,-6.76017690617));
#96294=CARTESIAN_POINT('Origin',(3.29394702409,-25.9742356128,-8.53006468251));
#96295=CARTESIAN_POINT('',(3.29394702904934,-26.2742356235235,-9.11457262156164));
#96296=CARTESIAN_POINT('Ctrl Pts',(3.59394702409,-25.9742356128,-8.84845722572));
#96297=CARTESIAN_POINT('Ctrl Pts',(3.59394702409,-25.9891777812359,-8.84845722572));
#96298=CARTESIAN_POINT('Ctrl Pts',(3.59282636130367,-26.0041057621838,-8.84954173138075));
#96299=CARTESIAN_POINT('Ctrl Pts',(3.59061714062251,-26.0188096181909,-8.85162544826636));
#96300=CARTESIAN_POINT('Ctrl Pts',(3.58839889516404,-26.0335735401874,-8.85371767723999));
#96301=CARTESIAN_POINT('Ctrl Pts',(3.58508344995202,-26.0481106067043,-8.85681729776892));
#96302=CARTESIAN_POINT('Ctrl Pts',(3.58075367323913,-26.0622239415934,-8.86083796584521));
#96303=CARTESIAN_POINT('Ctrl Pts',(3.57642912096537,-26.076320246907,-8.86485378246217));
#96304=CARTESIAN_POINT('Ctrl Pts',(3.57109322753218,-26.089993101306,-8.86978842524));
#96305=CARTESIAN_POINT('Ctrl Pts',(3.56487248323579,-26.1030742544672,-8.87555586234964));
#96306=CARTESIAN_POINT('Ctrl Pts',(3.55765481797495,-26.1182517606055,-8.88224757454468));
#96307=CARTESIAN_POINT('Ctrl Pts',(3.54924347424757,-26.1326432914629,-8.89002062963786));
#96308=CARTESIAN_POINT('Ctrl Pts',(3.53984316918362,-26.146093361616,-8.89865624715161));
#96309=CARTESIAN_POINT('Ctrl Pts',(3.53668269397923,-26.1506154077546,-8.90155962686548));
#96310=CARTESIAN_POINT('Ctrl Pts',(3.53341058644801,-26.1550314449506,-8.90456050810524));
#96311=CARTESIAN_POINT('Ctrl Pts',(3.53003502635557,-26.1593368153522,-8.90765057629916));
#96312=CARTESIAN_POINT('Ctrl Pts',(3.51871962783149,-26.1737690815695,-8.91800896190725));
#96313=CARTESIAN_POINT('Ctrl Pts',(3.50623880909602,-26.1869592376811,-8.92936841135558));
#96314=CARTESIAN_POINT('Ctrl Pts',(3.49286605549448,-26.1988045753596,-8.94144488155553));
#96315=CARTESIAN_POINT('Ctrl Pts',(3.48991429740156,-26.2014191880563,-8.9441105119641));
#96316=CARTESIAN_POINT('Ctrl Pts',(3.48691903007162,-26.2039684749351,-8.94681107663402));
#96317=CARTESIAN_POINT('Ctrl Pts',(3.48388309834292,-26.206451649493,-8.9495435208975));
#96318=CARTESIAN_POINT('Ctrl Pts',(3.46840744838,-26.2191096219669,-8.96347214470841));
#96319=CARTESIAN_POINT('Ctrl Pts',(3.45187175831933,-26.2300517991658,-8.97823314593818));
#96320=CARTESIAN_POINT('Ctrl Pts',(3.43460513144561,-26.2392173043093,-8.99349336029075));
#96321=CARTESIAN_POINT('Ctrl Pts',(3.43258777506472,-26.240288161427,-8.99527629629922));
#96322=CARTESIAN_POINT('Ctrl Pts',(3.43056040052516,-26.2413348070526,-8.99706604684286));
#96323=CARTESIAN_POINT('Ctrl Pts',(3.42852350169025,-26.2423571741797,-8.99886208056783));
#96324=CARTESIAN_POINT('Ctrl Pts',(3.40860261656626,-26.2523559319703,-9.01642730319981));
#96325=CARTESIAN_POINT('Ctrl Pts',(3.38776498003673,-26.2600351445809,-9.03460259281844));
#96326=CARTESIAN_POINT('Ctrl Pts',(3.36643491858791,-26.2653464252946,-9.05297755580061));
#96327=CARTESIAN_POINT('Ctrl Pts',(3.34271095817104,-26.2712537975596,-9.07341476342406));
#96328=CARTESIAN_POINT('Ctrl Pts',(3.31836689102333,-26.2742356128,-9.09410743824334));
#96329=CARTESIAN_POINT('Ctrl Pts',(3.29394702409,-26.2742356128,-9.11457260736));
#96330=CARTESIAN_POINT('',(3.29394702409,-26.2742356128,-6.76017690617));
#96331=CARTESIAN_POINT('',(3.29394702409,-26.2742356128,-8.43254284669));
#96332=CARTESIAN_POINT('Origin',(3.29394702409,-25.9742356128,-6.76017690617));
#96333=CARTESIAN_POINT('Origin',(-2.68618205273E-16,-26.2742356128,0.729452270839));
#96334=CARTESIAN_POINT('',(-3.29394702409,-26.2742356128,-9.11457265181));
#96335=CARTESIAN_POINT('',(-3.29394702409,-26.2742356128,-6.76017690617));
#96336=CARTESIAN_POINT('',(-3.29394702409,-26.2742356128,-8.53006468251));
#96337=CARTESIAN_POINT('',(-0.728014505146,-26.2742356128,-7.7348985358));
#96338=CARTESIAN_POINT('Origin',(2.84607155346,-26.2742356128,5.53854202767));
#96339=CARTESIAN_POINT('',(0.728014505146,-26.2742356128,-7.7348985358));
#96340=CARTESIAN_POINT('Origin',(1.52421666678E-14,-26.2742356128,-5.03119831567));
#96341=CARTESIAN_POINT('Origin',(-2.84607155346,-26.2742356128,5.53854202767));
#96342=CARTESIAN_POINT('',(0.582701491963,-26.2742356128,-9.97458510214));
#96343=CARTESIAN_POINT('Origin',(-2.84607155346,-26.2742356128,5.53854202767));
#96344=CARTESIAN_POINT('',(-0.582701491963,-26.2742356128,-9.97458510214));
#96345=CARTESIAN_POINT('Origin',(2.04045674064E-15,-26.2742356128,-7.33821278943));
#96346=CARTESIAN_POINT('Origin',(2.84607155346,-26.2742356128,5.53854202767));
#96347=CARTESIAN_POINT('Origin',(3.29394702409,-24.7242356128,-6.76017690617));
#96348=CARTESIAN_POINT('',(3.15994605614,-23.4742356128,-6.49176725547));
#96349=CARTESIAN_POINT('Origin',(3.29394702409,-23.4742356128,-6.76017690617));
#96350=CARTESIAN_POINT('',(3.15994605614,-25.9742356128,-6.49176725547));
#96351=CARTESIAN_POINT('Origin',(3.29394702409,-25.9742356128,-6.76017690617));
#96352=CARTESIAN_POINT('',(3.15994605614,-24.7267356128,-6.49176725547));
#96353=CARTESIAN_POINT('Origin',(3.29394702409,-25.9742356128,-6.76017690617));
#96354=CARTESIAN_POINT('Origin',(3.29394702409,-25.9742356128,-6.76017690617));
#96355=CARTESIAN_POINT('Origin',(-2.84607155346,-25.9742356128,5.53854202767));
#96356=CARTESIAN_POINT('',(0.650012951023,-25.9742356128,-7.44521636936));
#96357=CARTESIAN_POINT('Origin',(-2.84607155346,-25.9742356128,5.53854202767));
#96358=CARTESIAN_POINT('Origin',(0.728014505146,-25.9742356128,-7.7348985358));
#96359=CARTESIAN_POINT('Origin',(-2.84607155346,-24.4742356128,5.53854202767));
#96360=CARTESIAN_POINT('',(0.650012951023,-23.4742356128,-7.44521636936));
#96361=CARTESIAN_POINT('',(0.650012951023,-24.7267356128,-7.44521636936));
#96362=CARTESIAN_POINT('Origin',(-2.84607155346,-23.4742356128,5.53854202767));
#96363=CARTESIAN_POINT('Origin',(1.52789060718E-14,-25.9742356128,-5.03119831567));
#96364=CARTESIAN_POINT('',(-0.650012951023,-25.9742356128,-7.44521636936));
#96365=CARTESIAN_POINT('Origin',(1.55009506767E-14,-25.9742356128,-5.03119831567));
#96366=CARTESIAN_POINT('Origin',(-0.728014505146,-25.9742356128,-7.7348985358));
#96367=CARTESIAN_POINT('Origin',(1.56846476966E-14,-24.4742356128,-5.03119831567));
#96368=CARTESIAN_POINT('',(-0.650012951023,-23.4742356128,-7.44521636936));
#96369=CARTESIAN_POINT('',(-0.650012951023,-24.7267356128,-7.44521636936));
#96370=CARTESIAN_POINT('Origin',(1.60291569814E-14,-23.4742356128,-5.03119831567));
#96371=CARTESIAN_POINT('Origin',(2.84607155346,-25.9742356128,5.53854202767));
#96372=CARTESIAN_POINT('',(-3.15994605614,-25.9742356128,-6.49176725547));
#96373=CARTESIAN_POINT('Origin',(2.84607155346,-25.9742356128,5.53854202767));
#96374=CARTESIAN_POINT('Origin',(-3.29394702409,-25.9742356128,-6.76017690617));
#96375=CARTESIAN_POINT('Origin',(2.84607155346,-24.4742356128,5.53854202767));
#96376=CARTESIAN_POINT('',(-3.15994605614,-23.4742356128,-6.49176725547));
#96377=CARTESIAN_POINT('',(-3.15994605614,-24.7242356128,-6.49176725547));
#96378=CARTESIAN_POINT('Origin',(2.84607155346,-23.4742356128,5.53854202767));
#96379=CARTESIAN_POINT('Origin',(-3.29394702409,-25.9742356128,-8.53006468251));
#96380=CARTESIAN_POINT('',(-3.59394702409,-25.9742356128,-8.84845722568));
#96381=CARTESIAN_POINT('Ctrl Pts',(-3.29394702409,-26.2742356128,-9.11457265181));
#96382=CARTESIAN_POINT('Ctrl Pts',(-3.30720704925,-26.2742356128,-9.1034600928));
#96383=CARTESIAN_POINT('Ctrl Pts',(-3.32044878803,-26.2735029951,-9.09229236737));
#96384=CARTESIAN_POINT('Ctrl Pts',(-3.33363103946,-26.2720418371,-9.0811040513));
#96385=CARTESIAN_POINT('Ctrl Pts',(-3.37291095474,-26.2654802717,-9.04755646576));
#96386=CARTESIAN_POINT('Ctrl Pts',(-3.41093514101,-26.2524263623,-9.01447547571));
#96387=CARTESIAN_POINT('Ctrl Pts',(-3.43541561624,-26.240866543,-8.99291668586));
#96388=CARTESIAN_POINT('Ctrl Pts',(-3.46997146608,-26.219486164,-8.96214399258));
#96389=CARTESIAN_POINT('Ctrl Pts',(-3.50089098302,-26.1920639406,-8.9342126496));
#96390=CARTESIAN_POINT('Ctrl Pts',(-3.51056331552,-26.1824628447,-8.9254339626));
#96391=CARTESIAN_POINT('Ctrl Pts',(-3.52866003196,-26.1623189549,-8.90893921363));
#96392=CARTESIAN_POINT('Ctrl Pts',(-3.54462619729,-26.1398775942,-8.89427266222));
#96393=CARTESIAN_POINT('Ctrl Pts',(-3.55192119026,-26.1282916208,-8.88754705425));
#96394=CARTESIAN_POINT('Ctrl Pts',(-3.56506382466,-26.1044831752,-8.87539313986));
#96395=CARTESIAN_POINT('Ctrl Pts',(-3.57557442716,-26.0789471162,-8.86562061849));
#96396=CARTESIAN_POINT('Ctrl Pts',(-3.58006361288,-26.0660011409,-8.8614367189));
#96397=CARTESIAN_POINT('Ctrl Pts',(-3.58736522612,-26.0402449423,-8.8546203727));
#96398=CARTESIAN_POINT('Ctrl Pts',(-3.59178640039,-26.0136034223,-8.85048167902));
#96399=CARTESIAN_POINT('Ctrl Pts',(-3.59322678156,-26.0005307527,-8.8491320671));
#96400=CARTESIAN_POINT('Ctrl Pts',(-3.59394702493,-25.9873832723,-8.84845722511));
#96401=CARTESIAN_POINT('Ctrl Pts',(-3.59394702409,-25.9742356128,-8.84845722568));
#96402=CARTESIAN_POINT('',(-3.59394702409,-25.9742356128,-6.76017690617));
#96403=CARTESIAN_POINT('',(-3.59394702409,-25.9742356128,-7.89543489424));
#96404=CARTESIAN_POINT('Origin',(-3.29394702409,-25.9742356128,-6.76017690617));
#96405=CARTESIAN_POINT('Origin',(-3.29394702409,-25.9742356128,-6.76017690617));
#96406=CARTESIAN_POINT('Origin',(-3.29394702409,-25.9742356128,-6.76017690617));
#96407=CARTESIAN_POINT('Origin',(-3.29394702409,-24.7242356128,-6.76017690617));
#96408=CARTESIAN_POINT('',(-3.59394702409,-23.4742356128,-6.76017690617));
#96409=CARTESIAN_POINT('Origin',(-3.29394702409,-23.4742356128,-6.76017690617));
#96410=CARTESIAN_POINT('',(-3.59394702409,-24.7267356128,-6.76017690617));
#96411=CARTESIAN_POINT('Origin',(-3.59394702409,-23.1742356128,-9.19678210318));
#96412=CARTESIAN_POINT('',(-3.59394702409,-23.4742356128,-8.84845722572));
#96413=CARTESIAN_POINT('',(-3.59394702409,-27.9742356128,-8.84845722572));
#96414=CARTESIAN_POINT('',(-3.59394702409,-23.4742356128,3.49118372723));
#96415=CARTESIAN_POINT('Origin',(-1.02789922074E-15,-32.4742356128,0.729452270839));
#96416=CARTESIAN_POINT('',(12.4158605957,-32.4742356128,10.1688562115));
#96417=CARTESIAN_POINT('',(-12.4158605957,-32.4742356128,10.1688562115));
#96418=CARTESIAN_POINT('Origin',(-9.91308936055E-16,-32.4742356128,0.580061096523));
#96419=CARTESIAN_POINT('',(-12.9732844032,-32.4742356128,8.9713386779));
#96420=CARTESIAN_POINT('Origin',(-10.0415172382,-32.4742356128,8.33514586886));
#96421=CARTESIAN_POINT('',(-0.647446102181,-32.4742356128,-10.2675153591));
#96422=CARTESIAN_POINT('Origin',(2.84607155346,-32.4742356128,5.53854202767));
#96423=CARTESIAN_POINT('',(0.647446102181,-32.4742356128,-10.2675153591));
#96424=CARTESIAN_POINT('Origin',(9.48108817785E-16,-32.4742356128,-7.33821278943));
#96425=CARTESIAN_POINT('',(12.9732844032,-32.4742356128,8.9713386779));
#96426=CARTESIAN_POINT('Origin',(-2.84607155346,-32.4742356128,5.53854202767));
#96427=CARTESIAN_POINT('Origin',(10.0415172382,-32.4742356128,8.33514586886));
#96428=CARTESIAN_POINT('Origin',(-3.3774316049,-23.4742356128,-0.216889913236));
#96429=CARTESIAN_POINT('',(-12.7692410021,-23.1742356128,8.46695657076));
#96430=CARTESIAN_POINT('Origin',(-12.7692410021,-23.4742356128,8.46695657076));
#96431=CARTESIAN_POINT('',(-11.8109248062,-23.1742356128,7.5808790988));
#96432=CARTESIAN_POINT('Origin',(-11.8109248062,-23.4742356128,7.5808790988));
#96433=CARTESIAN_POINT('',(-12.2900829041,-23.1742356128,8.02391783478));
#96434=CARTESIAN_POINT('Origin',(-11.4035900518,-23.4742356128,8.02142239733));
#96435=CARTESIAN_POINT('',(-10.9011091428,-23.1742356128,7.69353074443));
#96436=CARTESIAN_POINT('Origin',(-10.9011091428,-23.4742356128,7.69353074443));
#96437=CARTESIAN_POINT('Origin',(-11.4035900518,-23.1742356128,8.02142239733));
#96438=CARTESIAN_POINT('Origin',(-3.36399067654E-14,-23.4742356128,0.580061096522));
#96439=CARTESIAN_POINT('',(-7.55300678542,-23.1742356128,11.1813685383));
#96440=CARTESIAN_POINT('Origin',(-7.55300678542,-23.4742356128,11.1813685383));
#96441=CARTESIAN_POINT('Origin',(-3.36841676743E-14,-23.1742356128,0.580061096522));
#96442=CARTESIAN_POINT('Origin',(-7.90115867216,-23.4742356128,11.6700302451));
#96443=CARTESIAN_POINT('',(-7.49382391778,-23.1742356128,12.1105735437));
#96444=CARTESIAN_POINT('Origin',(-7.49382391778,-23.4742356128,12.1105735437));
#96445=CARTESIAN_POINT('Origin',(-7.90115867216,-23.1742356128,11.6700302451));
#96446=CARTESIAN_POINT('Origin',(0.59766294349,-23.4742356128,4.62903013076));
#96447=CARTESIAN_POINT('',(-8.72866611926,-23.1742356128,13.252332246));
#96448=CARTESIAN_POINT('Origin',(-8.72866611926,-23.4742356128,13.252332246));
#96449=CARTESIAN_POINT('',(-8.11124501852,-23.1742356128,12.6814528948));
#96450=CARTESIAN_POINT('Origin',(-0.612454553411,-23.4742356128,4.61535352549));
#96451=CARTESIAN_POINT('',(8.72866611926,-23.1742356128,13.252332246));
#96452=CARTESIAN_POINT('Origin',(8.72866611926,-23.4742356128,13.252332246));
#96453=CARTESIAN_POINT('',(7.49382391778,-23.1742356128,12.1105735437));
#96454=CARTESIAN_POINT('Origin',(7.49382391778,-23.4742356128,12.1105735437));
#96455=CARTESIAN_POINT('',(8.11124501852,-23.1742356128,12.6814528948));
#96456=CARTESIAN_POINT('Origin',(7.90115867216,-23.4742356128,11.6700302451));
#96457=CARTESIAN_POINT('Origin',(7.90115867216,-23.1742356128,11.6700302451));
#96458=CARTESIAN_POINT('Origin',(11.4035900518,-23.4742356128,8.02142239733));
#96459=CARTESIAN_POINT('',(11.8109248062,-23.1742356128,7.5808790988));
#96460=CARTESIAN_POINT('Origin',(11.8109248062,-23.4742356128,7.5808790988));
#96461=CARTESIAN_POINT('Origin',(11.4035900518,-23.1742356128,8.02142239733));
#96462=CARTESIAN_POINT('Origin',(3.46618126442,-23.4742356128,-0.134830281674));
#96463=CARTESIAN_POINT('',(12.7692410021,-23.1742356128,8.46695657076));
#96464=CARTESIAN_POINT('Origin',(12.7692410021,-23.4742356128,8.46695657076));
#96465=CARTESIAN_POINT('',(12.2900829041,-23.1742356128,8.02391783478));
#96466=CARTESIAN_POINT('Origin',(3.89394702409,-23.4742356128,3.49118372723));
#96467=CARTESIAN_POINT('',(3.89394702409,-23.1742356128,-6.76017690617));
#96468=CARTESIAN_POINT('Origin',(3.89394702409,-23.4742356128,-6.76017690617));
#96469=CARTESIAN_POINT('',(3.89394702409,-23.1742356128,-8.84845722572));
#96470=CARTESIAN_POINT('',(3.89394702409,-23.1742356128,-7.80431706594));
#96471=CARTESIAN_POINT('Origin',(3.89394702409,-23.4742356128,-8.84845722572));
#96472=CARTESIAN_POINT('Origin',(3.29394702409,-23.4742356128,-6.76017690617));
#96473=CARTESIAN_POINT('',(3.02594508819,-23.1742356128,-6.22335760477));
#96474=CARTESIAN_POINT('Origin',(3.02594508819,-23.4742356128,-6.22335760477));
#96475=CARTESIAN_POINT('Origin',(3.29394702409,-23.1742356128,-6.76017690617));
#96476=CARTESIAN_POINT('Origin',(-2.84607155346,-23.4742356128,5.53854202767));
#96477=CARTESIAN_POINT('',(0.572011396901,-23.1742356128,-7.15553420291));
#96478=CARTESIAN_POINT('Origin',(0.572011396901,-23.4742356128,-7.15553420291));
#96479=CARTESIAN_POINT('Origin',(-2.84607155346,-23.1742356128,5.53854202767));
#96480=CARTESIAN_POINT('Origin',(1.60291569814E-14,-23.4742356128,-5.03119831567));
#96481=CARTESIAN_POINT('',(-0.572011396901,-23.1742356128,-7.15553420291));
#96482=CARTESIAN_POINT('Origin',(-0.572011396901,-23.4742356128,-7.15553420291));
#96483=CARTESIAN_POINT('Origin',(1.6213480319E-14,-23.1742356128,-5.03119831567));
#96484=CARTESIAN_POINT('Origin',(2.84607155346,-23.4742356128,5.53854202767));
#96485=CARTESIAN_POINT('',(-3.02594508819,-23.1742356128,-6.22335760477));
#96486=CARTESIAN_POINT('Origin',(-3.02594508819,-23.4742356128,-6.22335760477));
#96487=CARTESIAN_POINT('Origin',(2.84607155346,-23.1742356128,5.53854202767));
#96488=CARTESIAN_POINT('Origin',(-3.29394702409,-23.4742356128,-6.76017690617));
#96489=CARTESIAN_POINT('',(-3.89394702409,-23.1742356128,-6.76017690617));
#96490=CARTESIAN_POINT('Origin',(-3.89394702409,-23.4742356128,-6.76017690617));
#96491=CARTESIAN_POINT('Origin',(-3.29394702409,-23.1742356128,-6.76017690617));
#96492=CARTESIAN_POINT('Origin',(-3.89394702409,-23.4742356128,3.49118372723));
#96493=CARTESIAN_POINT('',(-3.89394702409,-23.1742356128,-8.84845722572));
#96494=CARTESIAN_POINT('Origin',(-3.89394702409,-23.4742356128,-8.84845722572));
#96495=CARTESIAN_POINT('',(-3.89394702409,-23.1742356128,-7.80431706594));
#96496=CARTESIAN_POINT('Origin',(1.11022302463E-16,-23.1742356128,0.729452270839));
#96497=CARTESIAN_POINT('Origin',(-2.84607155346,-23.1742356128,5.53854202767));
#96498=CARTESIAN_POINT('Origin',(2.84607155346,-23.1742356128,5.53854202767));
#96499=CARTESIAN_POINT('Origin',(5.47668310535E-15,-23.1742356128,0.580061096523));
#96500=CARTESIAN_POINT('Origin',(12.7692410021,-23.4742356128,8.46695657076));
#96501=CARTESIAN_POINT('',(13.0641007993,-23.4742356128,8.52225304435));
#96502=CARTESIAN_POINT('Origin',(12.7692410021,-23.4742356128,8.46695657076));
#96503=CARTESIAN_POINT('Origin',(12.7692410021,-23.4742356128,8.46695657076));
#96504=CARTESIAN_POINT('',(12.8356936926466,-23.1882133320383,8.52839999861852));
#96505=CARTESIAN_POINT('Origin',(12.7692410021,-23.4742356128,8.46695657076));
#96506=CARTESIAN_POINT('Origin',(3.89394702409,-23.4742356128,-8.84845722572));
#96507=CARTESIAN_POINT('',(4.02121700373,-23.4742356128,-9.12012310927));
#96508=CARTESIAN_POINT('Origin',(3.89394702409,-23.4742356128,-8.84845722572));
#96509=CARTESIAN_POINT('',(3.89394702409,-23.4742356128,-9.14845722572));
#96510=CARTESIAN_POINT('Origin',(3.89394702409,-23.4742356128,-8.84845722572));
#96511=CARTESIAN_POINT('',(3.89394702409,-23.4034955956937,-9.13999770314947));
#96512=CARTESIAN_POINT('Origin',(3.89394702409,-23.4742356128,-8.84845722572));
#96513=CARTESIAN_POINT('Origin',(3.89394702409,-23.4742356128,-8.84845722572));
#96514=CARTESIAN_POINT('Origin',(-2.84607155346,-23.4742356128,5.53854202767));
#96515=CARTESIAN_POINT('Origin',(-2.84607155346,-23.4742356128,5.53854202767));
#96516=CARTESIAN_POINT('Ctrl Pts',(12.5655736249,-25.9742356128,8.68722822002));
#96517=CARTESIAN_POINT('Ctrl Pts',(12.6125281896,-25.9742356128,8.73064330802));
#96518=CARTESIAN_POINT('Ctrl Pts',(12.6710473074,-25.9742356128,8.76156013382));
#96519=CARTESIAN_POINT('Ctrl Pts',(12.7367182007,-25.9742356128,8.77578329688));
#96520=CARTESIAN_POINT('Ctrl Pts',(12.8688414275,-25.9742356128,8.7679322687));
#96521=CARTESIAN_POINT('Ctrl Pts',(12.9795662208,-25.9742356128,8.69541878151));
#96522=CARTESIAN_POINT('Ctrl Pts',(13.0237889047,-25.9742356128,8.64482907085));
#96523=CARTESIAN_POINT('Ctrl Pts',(13.0523134365,-25.9742356128,8.58510731301));
#96524=CARTESIAN_POINT('Ctrl Pts',(13.0641007993,-25.9742356128,8.52225304435));
#96525=CARTESIAN_POINT('Ctrl Pts',(12.5655736249,-26.0156901503,8.68722822002));
#96526=CARTESIAN_POINT('Ctrl Pts',(12.6125281896,-26.0101392553,8.73064330802));
#96527=CARTESIAN_POINT('Ctrl Pts',(12.6710473074,-26.0069407531,8.76156013382));
#96528=CARTESIAN_POINT('Ctrl Pts',(12.7367182007,-26.0066348021,8.77578329688));
#96529=CARTESIAN_POINT('Ctrl Pts',(12.8688414275,-26.0118680127,8.7679322687));
#96530=CARTESIAN_POINT('Ctrl Pts',(12.9795662208,-26.0268285906,8.69541878151));
#96531=CARTESIAN_POINT('Ctrl Pts',(13.0237889047,-26.0362726342,8.64482907085));
#96532=CARTESIAN_POINT('Ctrl Pts',(13.0523134365,-26.0467091655,8.58510731301));
#96533=CARTESIAN_POINT('Ctrl Pts',(13.0641007993,-26.0571446878,8.52225304435));
#96534=CARTESIAN_POINT('Ctrl Pts',(12.5673190764,-26.0571611787,8.69860099886));
#96535=CARTESIAN_POINT('Ctrl Pts',(12.6147839704,-26.0460087182,8.73985554978));
#96536=CARTESIAN_POINT('Ctrl Pts',(12.6733623751,-26.039567434,8.7690990864));
#96537=CARTESIAN_POINT('Ctrl Pts',(12.7386568777,-26.038925371,8.78241060374));
#96538=CARTESIAN_POINT('Ctrl Pts',(12.8694529589,-26.0493679679,8.77449484918));
#96539=CARTESIAN_POINT('Ctrl Pts',(12.9783519251,-26.079330936,8.70501235676));
#96540=CARTESIAN_POINT('Ctrl Pts',(13.0216997747,-26.0982548482,8.65661829968));
#96541=CARTESIAN_POINT('Ctrl Pts',(13.0495520754,-26.1191713964,8.59946132904));
#96542=CARTESIAN_POINT('Ctrl Pts',(13.0609230524,-26.1400859332,8.53920080258));
#96543=CARTESIAN_POINT('Ctrl Pts',(12.5708020939,-26.0955898119,8.72129739555));
#96544=CARTESIAN_POINT('Ctrl Pts',(12.6192645611,-26.0807374464,8.75832152472));
#96545=CARTESIAN_POINT('Ctrl Pts',(12.6779437588,-26.072572542,8.78430344011));
#96546=CARTESIAN_POINT('Ctrl Pts',(12.7424767707,-26.0724883755,8.79585386213));
#96547=CARTESIAN_POINT('Ctrl Pts',(12.8706190688,-26.0884772207,8.78786373285));
#96548=CARTESIAN_POINT('Ctrl Pts',(12.9758918612,-26.1312493712,8.7243679619));
#96549=CARTESIAN_POINT('Ctrl Pts',(13.0175064499,-26.1580067779,8.68029613171));
#96550=CARTESIAN_POINT('Ctrl Pts',(13.0440297261,-26.1874767751,8.62818300551));
#96551=CARTESIAN_POINT('Ctrl Pts',(13.0545801486,-26.2169441965,8.57302387625));
#96552=CARTESIAN_POINT('Ctrl Pts',(12.5794459662,-26.1608028821,8.77948305254));
#96553=CARTESIAN_POINT('Ctrl Pts',(12.6296141113,-26.142770098,8.80804311593));
#96554=CARTESIAN_POINT('Ctrl Pts',(12.6879356315,-26.1342515256,8.82779050493));
#96555=CARTESIAN_POINT('Ctrl Pts',(12.7502196423,-26.1368008678,8.83632815809));
#96556=CARTESIAN_POINT('Ctrl Pts',(12.8715106952,-26.1635294701,8.82947566206));
#96557=CARTESIAN_POINT('Ctrl Pts',(12.9681422326,-26.2258042788,8.77959930959));
#96558=CARTESIAN_POINT('Ctrl Pts',(13.0057211957,-26.2639659335,8.74503645745));
#96559=CARTESIAN_POINT('Ctrl Pts',(13.0291938131,-26.3056693816,8.70391024913));
#96560=CARTESIAN_POINT('Ctrl Pts',(13.037895068,-26.3473699802,8.65987870015));
#96561=CARTESIAN_POINT('Ctrl Pts',(12.5904350881,-26.208935598,8.85843870903));
#96562=CARTESIAN_POINT('Ctrl Pts',(12.6413857281,-26.193073841,8.8794045658));
#96563=CARTESIAN_POINT('Ctrl Pts',(12.6981640128,-26.1879369487,8.89407137053));
#96564=CARTESIAN_POINT('Ctrl Pts',(12.7569188608,-26.1947558682,8.90085098743));
#96565=CARTESIAN_POINT('Ctrl Pts',(12.8688909488,-26.2311660085,8.89755364806));
#96566=CARTESIAN_POINT('Ctrl Pts',(12.9549222972,-26.3046245246,8.86341292137));
#96567=CARTESIAN_POINT('Ctrl Pts',(12.9876969697,-26.3485480349,8.83930386397));
#96568=CARTESIAN_POINT('Ctrl Pts',(13.0075899899,-26.3960930753,8.81007138323));
#96569=CARTESIAN_POINT('Ctrl Pts',(13.0141520182,-26.4436357412,8.77811343457));
#96570=CARTESIAN_POINT('Ctrl Pts',(12.5959177038,-26.2279044079,8.8994052873));
#96571=CARTESIAN_POINT('Ctrl Pts',(12.646874483,-26.2139581927,8.91740539891));
#96572=CARTESIAN_POINT('Ctrl Pts',(12.7025812771,-26.2109800213,8.93027129181));
#96573=CARTESIAN_POINT('Ctrl Pts',(12.7593862349,-26.2199914752,8.93670805691));
#96574=CARTESIAN_POINT('Ctrl Pts',(12.8665236815,-26.2605801567,8.93574094902));
#96575=CARTESIAN_POINT('Ctrl Pts',(12.9473429566,-26.3377051372,8.90908651151));
#96576=CARTESIAN_POINT('Ctrl Pts',(12.9777936856,-26.3833026499,8.88980176083));
#96577=CARTESIAN_POINT('Ctrl Pts',(12.9959671442,-26.4324389347,8.86600393028));
#96578=CARTESIAN_POINT('Ctrl Pts',(13.0015068071,-26.4815731476,8.83957127532));
#96579=CARTESIAN_POINT('Ctrl Pts',(12.6014286433,-26.242977575,8.94251399615));
#96580=CARTESIAN_POINT('Ctrl Pts',(12.6520390535,-26.231349296,8.95817349548));
#96581=CARTESIAN_POINT('Ctrl Pts',(12.7063906649,-26.2306858466,8.96978929718));
#96582=CARTESIAN_POINT('Ctrl Pts',(12.7610505563,-26.2417976368,8.97629178839));
#96583=CARTESIAN_POINT('Ctrl Pts',(12.8631123569,-26.2859464251,8.9781294015));
#96584=CARTESIAN_POINT('Ctrl Pts',(12.9386865297,-26.365438177,8.95883155382));
#96585=CARTESIAN_POINT('Ctrl Pts',(12.9668261506,-26.4119362845,8.94417302517));
#96586=CARTESIAN_POINT('Ctrl Pts',(12.9832936343,-26.4618287729,8.92554423077));
#96587=CARTESIAN_POINT('Ctrl Pts',(12.9878157168,-26.5117194744,8.90437404317));
#96588=CARTESIAN_POINT('Ctrl Pts',(12.606833891,-26.2541478224,8.98696694086));
#96589=CARTESIAN_POINT('Ctrl Pts',(12.6567634559,-26.2450231646,9.00090329165));
#96590=CARTESIAN_POINT('Ctrl Pts',(12.7095130326,-26.2466650943,9.01179180097));
#96591=CARTESIAN_POINT('Ctrl Pts',(12.7618789354,-26.2596853008,9.01872934487));
#96592=CARTESIAN_POINT('Ctrl Pts',(12.8587193341,-26.3067070888,9.02376000338));
#96593=CARTESIAN_POINT('Ctrl Pts',(12.9290963448,-26.3874138436,9.01159791107));
#96594=CARTESIAN_POINT('Ctrl Pts',(12.954969534,-26.4341563453,9.00132365176));
#96595=CARTESIAN_POINT('Ctrl Pts',(12.969765568,-26.4841089383,8.98755447916));
#96596=CARTESIAN_POINT('Ctrl Pts',(12.9732844047,-26.5340600059,8.97133867828));
#96597=CARTESIAN_POINT('',(13.0641007993,-25.9742356128,8.52225304435));
#96598=CARTESIAN_POINT('Origin',(12.7692410021,-25.9742356128,8.46695657076));
#96599=CARTESIAN_POINT('',(12.9732844000412,-26.5340599311358,8.97133869610266));
#96600=CARTESIAN_POINT('Origin',(12.6801075664532,-26.5340600708344,8.90771940054616));
#96601=CARTESIAN_POINT('Ctrl Pts',(13.0641007993,-25.9742356128,8.52225304435));
#96602=CARTESIAN_POINT('Ctrl Pts',(13.0641007993,-26.0571446878,8.52225304435));
#96603=CARTESIAN_POINT('Ctrl Pts',(13.0609230524,-26.1400859332,8.53920080258));
#96604=CARTESIAN_POINT('Ctrl Pts',(13.0545801486,-26.2169441965,8.57302387625));
#96605=CARTESIAN_POINT('Ctrl Pts',(13.037895068,-26.3473699802,8.65987870015));
#96606=CARTESIAN_POINT('Ctrl Pts',(13.0141520182,-26.4436357412,8.77811343457));
#96607=CARTESIAN_POINT('Ctrl Pts',(13.0015068071,-26.4815731476,8.83957127532));
#96608=CARTESIAN_POINT('Ctrl Pts',(12.9878157168,-26.5117194744,8.90437404317));
#96609=CARTESIAN_POINT('Ctrl Pts',(12.9732844047,-26.5340600059,8.97133867828));
#96610=CARTESIAN_POINT('Origin',(12.7692410021,-27.9742356128,8.46695657076));
#96611=CARTESIAN_POINT('',(13.0641007993,-27.8242356128,8.52225304435));
#96612=CARTESIAN_POINT('Origin',(3.89394702409,-27.9742356128,-8.84845722572));
#96613=CARTESIAN_POINT('',(4.02121700373,-25.9742356128,-9.12012310927));
#96614=CARTESIAN_POINT('',(4.02121700373,-27.8242356128,-9.12012310927));
#96615=CARTESIAN_POINT('Ctrl Pts',(3.59394702409,-25.9742356128,-8.84845722572));
#96616=CARTESIAN_POINT('Ctrl Pts',(3.59394702409,-25.9742356128002,-8.96899190619));
#96617=CARTESIAN_POINT('Ctrl Pts',(3.65448289574,-25.9742356128002,-9.08952658665));
#96618=CARTESIAN_POINT('Ctrl Pts',(3.77723460344,-25.9742356128002,-9.1675743146));
#96619=CARTESIAN_POINT('Ctrl Pts',(3.91206646884,-25.9742356128003,-9.17125793036));
#96620=CARTESIAN_POINT('Ctrl Pts',(4.02121700373,-25.9742356128,-9.12012310927));
#96621=CARTESIAN_POINT('Ctrl Pts',(4.02121700311545,-25.9742087333861,-9.12012310955797));
#96622=CARTESIAN_POINT('Ctrl Pts',(3.91205553437643,-25.9742146970064,-9.1712630529297));
#96623=CARTESIAN_POINT('Ctrl Pts',(3.77720758969876,-25.9742206606268,-9.1675735762));
#96624=CARTESIAN_POINT('Ctrl Pts',(3.65444600647237,-25.9742245217385,-9.089503129595));
#96625=CARTESIAN_POINT('Ctrl Pts',(3.5939227712474,-25.9742247028758,-8.96894360624986));
#96626=CARTESIAN_POINT('Ctrl Pts',(3.59394702986297,-25.9742221718257,-8.84839685399463));
#96627=CARTESIAN_POINT('Ctrl Pts',(4.02122205614958,-26.0847136525922,-9.12012074183368));
#96628=CARTESIAN_POINT('Ctrl Pts',(3.91205926363719,-26.0602023764211,-9.17126135222328));
#96629=CARTESIAN_POINT('Ctrl Pts',(3.77720986797824,-26.0356911001499,-9.16757232040782));
#96630=CARTESIAN_POINT('Ctrl Pts',(3.65444734645218,-26.0198214098812,-9.08950176074631));
#96631=CARTESIAN_POINT('Ctrl Pts',(3.5939243024794,-26.0190768988899,-8.96894175972539));
#96632=CARTESIAN_POINT('Ctrl Pts',(3.59394951005266,-26.029479841544,-8.84839452991358));
#96633=CARTESIAN_POINT('Ctrl Pts',(3.99525994980673,-26.1953560420414,-9.1322859303989));
#96634=CARTESIAN_POINT('Ctrl Pts',(3.89289863013481,-26.146162866449,-9.17999943960044));
#96635=CARTESIAN_POINT('Ctrl Pts',(3.76550434421357,-26.0969696909566,-9.17402461392749));
#96636=CARTESIAN_POINT('Ctrl Pts',(3.64756279207107,-26.065177481353,-9.09653482858758));
#96637=CARTESIAN_POINT('Ctrl Pts',(3.58605698027632,-26.0638115296301,-8.97842905062067));
#96638=CARTESIAN_POINT('Ctrl Pts',(3.58120648340124,-26.0848066822428,-8.86033548279754));
#96639=CARTESIAN_POINT('Ctrl Pts',(3.94360062276572,-26.293916292257,-9.15648299770932));
#96640=CARTESIAN_POINT('Ctrl Pts',(3.85442237244048,-26.2261168661153,-9.19756876089837));
#96641=CARTESIAN_POINT('Ctrl Pts',(3.7414986999235,-26.1583174399736,-9.18721517340115));
#96642=CARTESIAN_POINT('Ctrl Pts',(3.6330764351228,-26.1131686986625,-9.11086249079868));
#96643=CARTESIAN_POINT('Ctrl Pts',(3.56996718935291,-26.108201380164,-8.9974689177855));
#96644=CARTESIAN_POINT('Ctrl Pts',(3.55585088691963,-26.1340888379853,-8.88408647848547));
#96645=CARTESIAN_POINT('Ctrl Pts',(3.81878709152418,-26.4439556743499,-9.21381749055382));
#96646=CARTESIAN_POINT('Ctrl Pts',(3.75615830652382,-26.3530421884608,-9.24190779271982));
#96647=CARTESIAN_POINT('Ctrl Pts',(3.6725256492406,-26.2621287025717,-9.22341791384639));
#96648=CARTESIAN_POINT('Ctrl Pts',(3.58523528668288,-26.1982144741315,-9.14939448447646));
#96649=CARTESIAN_POINT('Ctrl Pts',(3.5232681863945,-26.1833159073178,-9.0448740837474));
#96650=CARTESIAN_POINT('Ctrl Pts',(3.49459357993615,-26.2091086215099,-8.94036284953103));
#96651=CARTESIAN_POINT('Ctrl Pts',(3.65518574680024,-26.5331576706117,-9.28645512724112));
#96652=CARTESIAN_POINT('Ctrl Pts',(3.62051284919576,-26.434977950602,-9.30153534977169));
#96653=CARTESIAN_POINT('Ctrl Pts',(3.56782721193058,-26.3367982306924,-9.27548347767736));
#96654=CARTESIAN_POINT('Ctrl Pts',(3.50535217434315,-26.263852978627,-9.20388490272889));
#96655=CARTESIAN_POINT('Ctrl Pts',(3.45109619805268,-26.2377244615336,-9.10776802330137));
#96656=CARTESIAN_POINT('Ctrl Pts',(3.41430468871176,-26.2537045861121,-9.01165851362097));
#96657=CARTESIAN_POINT('Ctrl Pts',(3.5753967783082,-26.560421829436,-9.32123386752726));
#96658=CARTESIAN_POINT('Ctrl Pts',(3.55290435767089,-26.46163192706,-9.33083686690438));
#96659=CARTESIAN_POINT('Ctrl Pts',(3.51371779768073,-26.3628420247839,-9.30175173243743));
#96660=CARTESIAN_POINT('Ctrl Pts',(3.46268894387028,-26.2877149808645,-9.23119412114871));
#96661=CARTESIAN_POINT('Ctrl Pts',(3.41348702446829,-26.2568846180366,-9.13849094265645));
#96662=CARTESIAN_POINT('Ctrl Pts',(3.37514906929817,-26.2673339290873,-9.04579442022087));
#96663=CARTESIAN_POINT('Ctrl Pts',(3.49280842183818,-26.5742388712317,-9.35651769670719));
#96664=CARTESIAN_POINT('Ctrl Pts',(3.48193300696612,-26.4768356794767,-9.36107471062541));
#96665=CARTESIAN_POINT('Ctrl Pts',(3.45560668553042,-26.3794324877216,-9.32929021973307));
#96666=CARTESIAN_POINT('Ctrl Pts',(3.41589189003752,-26.3038151487329,-9.25969681792774));
#96667=CARTESIAN_POINT('Ctrl Pts',(3.37274412802113,-26.2692830090117,-9.17005833196199));
#96668=CARTESIAN_POINT('Ctrl Pts',(3.33461993282405,-26.274239735331,-9.08042587139392));
#96669=CARTESIAN_POINT('Ctrl Pts',(3.40986370467272,-26.5742356882418,-9.39127343593685));
#96670=CARTESIAN_POINT('Ctrl Pts',(3.40986677190155,-26.4799793512239,-9.39127214064104));
#96671=CARTESIAN_POINT('Ctrl Pts',(3.39556373278484,-26.3857230142061,-9.35712926318368));
#96672=CARTESIAN_POINT('Ctrl Pts',(3.36677172202495,-26.3112263962281,-9.28841020083968));
#96673=CARTESIAN_POINT('Ctrl Pts',(3.33034394782978,-26.274222231551,-9.20147178423216));
#96674=CARTESIAN_POINT('Ctrl Pts',(3.29391705058738,-26.2742356584786,-9.11453884399441));
#96675=CARTESIAN_POINT('',(3.40988747183743,-26.5742356512186,-9.39126347679935));
#96676=CARTESIAN_POINT('Ctrl Pts',(4.02121700373,-25.9742356128,-9.12012310927));
#96677=CARTESIAN_POINT('Ctrl Pts',(4.02121700373,-26.0847351827,-9.12012310927));
#96678=CARTESIAN_POINT('Ctrl Pts',(3.99525241027,-26.1953704263,-9.13228946189));
#96679=CARTESIAN_POINT('Ctrl Pts',(3.94359404173,-26.2939242033,-9.15648602078));
#96680=CARTESIAN_POINT('Ctrl Pts',(3.81878605501,-26.4439540873,-9.2138179004));
#96681=CARTESIAN_POINT('Ctrl Pts',(3.65519433633,-26.5331529872,-9.28645131356));
#96682=CARTESIAN_POINT('Ctrl Pts',(3.57541049572,-26.560417142,-9.32122788832));
#96683=CARTESIAN_POINT('Ctrl Pts',(3.49282735343,-26.5742357037,-9.35650960864));
#96684=CARTESIAN_POINT('Ctrl Pts',(3.4098874718,-26.5742356887,-9.39126347671));
#96685=CARTESIAN_POINT('Origin',(3.29476705670924,-26.5721143469785,-9.11652908600206));
#96686=CARTESIAN_POINT('Origin',(-2.84607155346,-26.5742356128,5.53854202767));
#96687=CARTESIAN_POINT('',(0.647446102181,-26.5742356128,-10.2675153591));
#96688=CARTESIAN_POINT('Origin',(-2.84607155346,-26.5742356128,5.53854202767));
#96689=CARTESIAN_POINT('Origin',(0.582701491963,-26.5742356128,-9.97458510214));
#96690=CARTESIAN_POINT('Origin',(-2.84607155346,-27.8242356128,5.53854202767));
#96691=CARTESIAN_POINT('',(12.9732844032,-27.8242356128,8.9713386779));
#96692=CARTESIAN_POINT('',(0.647446102181,-27.8242356128,-10.2675153591));
#96693=CARTESIAN_POINT('Origin',(2.00371733667E-15,-26.5742356128,-7.33821278943));
#96694=CARTESIAN_POINT('',(-0.647446102181,-26.5742356128,-10.2675153591));
#96695=CARTESIAN_POINT('Origin',(1.67065042928E-15,-26.5742356128,-7.33821278943));
#96696=CARTESIAN_POINT('Origin',(-0.582701491963,-26.5742356128,-9.97458510214));
#96697=CARTESIAN_POINT('Origin',(1.51756957939E-15,-27.8242356128,-7.33821278943));
#96698=CARTESIAN_POINT('',(-0.647446102181,-27.8242356128,-10.2675153591));
#96699=CARTESIAN_POINT('Origin',(-12.7692410021,-23.4742356128,8.46695657076));
#96700=CARTESIAN_POINT('',(-13.0641007993,-23.4742356128,8.52225304435));
#96701=CARTESIAN_POINT('',(-12.9895126513631,-23.4742356128,8.67062394794872));
#96702=CARTESIAN_POINT('Origin',(-12.7692410021,-23.4742356128,8.46695657076));
#96703=CARTESIAN_POINT('',(-12.9840525338676,-23.4078536953505,8.66557541894761));
#96704=CARTESIAN_POINT('Origin',(-12.7692410021,-23.4742356128,8.46695657076));
#96705=CARTESIAN_POINT('Origin',(-12.7692410021,-23.4742356128,8.46695657076));
#96706=CARTESIAN_POINT('Origin',(-12.7692410021,-23.4742356128,8.46695657076));
#96707=CARTESIAN_POINT('Origin',(-3.89394702409,-23.4742356128,-8.84845722572));
#96708=CARTESIAN_POINT('',(-4.02121700373,-23.4742356128,-9.12012310927));
#96709=CARTESIAN_POINT('Origin',(-3.89394702409,-23.4742356128,-8.84845722572));
#96710=CARTESIAN_POINT('Origin',(-3.89394702409,-23.4742356128,-8.84845722572));
#96711=CARTESIAN_POINT('',(-3.89394702409,-23.1865648064703,-8.93357777074639));
#96712=CARTESIAN_POINT('Origin',(-3.89394702409,-23.4742356128,-8.84845722572));
#96713=CARTESIAN_POINT('Origin',(2.84607155346,-23.4742356128,5.53854202767));
#96714=CARTESIAN_POINT('Origin',(2.84607155346,-23.4742356128,5.53854202767));
#96715=CARTESIAN_POINT('Ctrl Pts',(-12.6068339386,-26.2541477285,8.98696689141));
#96716=CARTESIAN_POINT('Ctrl Pts',(-12.656763501,-26.2450230638,9.00090325616));
#96717=CARTESIAN_POINT('Ctrl Pts',(-12.7095130758,-26.2466649863,9.01179177872));
#96718=CARTESIAN_POINT('Ctrl Pts',(-12.7618789767,-26.2596851856,9.018729334));
#96719=CARTESIAN_POINT('Ctrl Pts',(-12.8587193698,-26.30670696,9.02376000973));
#96720=CARTESIAN_POINT('Ctrl Pts',(-12.9290963696,-26.3874137021,9.01159792233));
#96721=CARTESIAN_POINT('Ctrl Pts',(-12.9549695516,-26.4341561975,9.00132366206));
#96722=CARTESIAN_POINT('Ctrl Pts',(-12.9697655766,-26.4841087839,8.98755448534));
#96723=CARTESIAN_POINT('Ctrl Pts',(-12.9732844032,-26.5340598441,8.9713386779));
#96724=CARTESIAN_POINT('Ctrl Pts',(-12.602271199,-26.244718344,8.94944232356));
#96725=CARTESIAN_POINT('Ctrl Pts',(-12.6527754898,-26.2334802622,8.96483328464));
#96726=CARTESIAN_POINT('Ctrl Pts',(-12.7068774073,-26.2331761106,8.97633576006));
#96727=CARTESIAN_POINT('Ctrl Pts',(-12.761179757,-26.2445853283,8.98290608319));
#96728=CARTESIAN_POINT('Ctrl Pts',(-12.8624277437,-26.2891818679,8.98524139971));
#96729=CARTESIAN_POINT('Ctrl Pts',(-12.9371918658,-26.3688629587,8.96705573637));
#96730=CARTESIAN_POINT('Ctrl Pts',(-12.964978225,-26.4153991423,8.95308053464));
#96731=CARTESIAN_POINT('Ctrl Pts',(-12.9811851756,-26.4653009826,8.93520914846));
#96732=CARTESIAN_POINT('Ctrl Pts',(-12.9855508674,-26.5152010752,8.91481113395));
#96733=CARTESIAN_POINT('Ctrl Pts',(-12.5976340417,-26.2325138521,8.912882128));
#96734=CARTESIAN_POINT('Ctrl Pts',(-12.6484748874,-26.2192934199,8.93016638754));
#96735=CARTESIAN_POINT('Ctrl Pts',(-12.7037532053,-26.2170356489,8.94265428589));
#96736=CARTESIAN_POINT('Ctrl Pts',(-12.7598856352,-26.2266967758,8.94911991702));
#96737=CARTESIAN_POINT('Ctrl Pts',(-12.8654365701,-26.2683789496,8.94903642348));
#96738=CARTESIAN_POINT('Ctrl Pts',(-12.9446209623,-26.3462161918,8.92467166475));
#96739=CARTESIAN_POINT('Ctrl Pts',(-12.9743518533,-26.3920801662,8.90682449267));
#96740=CARTESIAN_POINT('Ctrl Pts',(-12.9919939688,-26.4414371519,8.88463204637));
#96741=CARTESIAN_POINT('Ctrl Pts',(-12.9972165276,-26.4907921504,8.8598339424));
#96742=CARTESIAN_POINT('Ctrl Pts',(-12.5930010467,-26.2175177033,8.87774657721));
#96743=CARTESIAN_POINT('Ctrl Pts',(-12.6439314611,-26.2025806566,8.89736399926));
#96744=CARTESIAN_POINT('Ctrl Pts',(-12.7001900362,-26.1984644898,8.91122227553));
#96745=CARTESIAN_POINT('Ctrl Pts',(-12.7580199858,-26.2063019338,8.91786661014));
#96746=CARTESIAN_POINT('Ctrl Pts',(-12.8677144157,-26.2446206613,8.91568901553));
#96747=CARTESIAN_POINT('Ctrl Pts',(-12.9513046343,-26.319697988,8.88504420709));
#96748=CARTESIAN_POINT('Ctrl Pts',(-12.982992513,-26.3643472171,8.86318110532));
#96749=CARTESIAN_POINT('Ctrl Pts',(-13.002081513,-26.4125746646,8.83647618314));
#96750=CARTESIAN_POINT('Ctrl Pts',(-13.0081651461,-26.4607998779,8.80708839192));
#96751=CARTESIAN_POINT('Ctrl Pts',(-12.5818292035,-26.1733614649,8.79590968998));
#96752=CARTESIAN_POINT('Ctrl Pts',(-12.6323244128,-26.1554842052,8.82249979162));
#96753=CARTESIAN_POINT('Ctrl Pts',(-12.6904347476,-26.1475299818,8.84085890335));
#96754=CARTESIAN_POINT('Ctrl Pts',(-12.7520318679,-26.1509983382,8.84880669813));
#96755=CARTESIAN_POINT('Ctrl Pts',(-12.8713824144,-26.1801158283,8.84250417641));
#96756=CARTESIAN_POINT('Ctrl Pts',(-12.9656920029,-26.2455948371,8.79617037266));
#96757=CARTESIAN_POINT('Ctrl Pts',(-13.0022038566,-26.2854891551,8.76401868675));
#96758=CARTESIAN_POINT('Ctrl Pts',(-13.0248773755,-26.3289895549,8.72565667529));
#96759=CARTESIAN_POINT('Ctrl Pts',(-13.0330999298,-26.3724871935,8.68442780782));
#96760=CARTESIAN_POINT('Ctrl Pts',(-12.5723981851,-26.1119182248,8.73171604256));
#96761=CARTESIAN_POINT('Ctrl Pts',(-12.6212992155,-26.0956425018,8.76686070247));
#96762=CARTESIAN_POINT('Ctrl Pts',(-12.6800096167,-26.086872764,8.79140324302));
#96763=CARTESIAN_POINT('Ctrl Pts',(-12.7441850222,-26.0871118638,8.8021873834));
#96764=CARTESIAN_POINT('Ctrl Pts',(-12.8711063426,-26.1055282096,8.79420158155));
#96765=CARTESIAN_POINT('Ctrl Pts',(-12.9747302188,-26.1536338998,8.73340720985));
#96766=CARTESIAN_POINT('Ctrl Pts',(-13.0155596279,-26.1836251588,8.69127581187));
#96767=CARTESIAN_POINT('Ctrl Pts',(-13.0414826419,-26.2166144707,8.64142369403));
#96768=CARTESIAN_POINT('Ctrl Pts',(-13.0516641058,-26.249601018,8.58855181802));
#96769=CARTESIAN_POINT('Ctrl Pts',(-12.5678634067,-26.0691543106,8.70214065489));
#96770=CARTESIAN_POINT('Ctrl Pts',(-12.6154947189,-26.0563582708,8.74269816246));
#96771=CARTESIAN_POINT('Ctrl Pts',(-12.6740974841,-26.0489588063,8.77139810866));
#96772=CARTESIAN_POINT('Ctrl Pts',(-12.7392779978,-26.0482057465,8.7844092739));
#96773=CARTESIAN_POINT('Ctrl Pts',(-12.8696620869,-26.0601436152,8.77645823375));
#96774=CARTESIAN_POINT('Ctrl Pts',(-12.9779865573,-26.0944629325,8.70793763124));
#96775=CARTESIAN_POINT('Ctrl Pts',(-13.0210579562,-26.1161437068,8.66024422424));
#96776=CARTESIAN_POINT('Ctrl Pts',(-13.0486971014,-26.140109634,8.6039070082));
#96777=CARTESIAN_POINT('Ctrl Pts',(-13.0599353737,-26.1640732171,8.54447530783));
#96778=CARTESIAN_POINT('Ctrl Pts',(-12.5655736321,-26.0216427322,8.68722826989));
#96779=CARTESIAN_POINT('Ctrl Pts',(-12.6125281998,-26.0152947619,8.73064336108));
#96780=CARTESIAN_POINT('Ctrl Pts',(-12.6710473198,-26.011636969,8.76156019108));
#96781=CARTESIAN_POINT('Ctrl Pts',(-12.7367182138,-26.0112870749,8.77578335878));
#96782=CARTESIAN_POINT('Ctrl Pts',(-12.8688414379,-26.0172717145,8.76793233964));
#96783=CARTESIAN_POINT('Ctrl Pts',(-12.9795662207,-26.0343805031,8.69541885992));
#96784=CARTESIAN_POINT('Ctrl Pts',(-13.0237888974,-26.0451806345,8.64482915231));
#96785=CARTESIAN_POINT('Ctrl Pts',(-13.0523134203,-26.0571157701,8.58510739684));
#96786=CARTESIAN_POINT('Ctrl Pts',(-13.0641007736,-26.0690497547,8.52225313007));
#96787=CARTESIAN_POINT('Ctrl Pts',(-12.5655736251,-25.9742356164,8.68722820936));
#96788=CARTESIAN_POINT('Ctrl Pts',(-12.6125281889,-25.9742356185,8.7306432957));
#96789=CARTESIAN_POINT('Ctrl Pts',(-12.6710473059,-25.974235622,8.76156011981));
#96790=CARTESIAN_POINT('Ctrl Pts',(-12.7367181986,-25.9742356268,8.7757832814));
#96791=CARTESIAN_POINT('Ctrl Pts',(-12.8688414249,-25.9742356378,8.76793225111));
#96792=CARTESIAN_POINT('Ctrl Pts',(-12.97956622,-25.9742356495,8.6954187635));
#96793=CARTESIAN_POINT('Ctrl Pts',(-13.0237889055,-25.9742356551,8.64482905307));
#96794=CARTESIAN_POINT('Ctrl Pts',(-13.0523134395,-25.9742356597,8.58510729574));
#96795=CARTESIAN_POINT('Ctrl Pts',(-13.0641008049,-25.9742356631,8.52225302769));
#96796=CARTESIAN_POINT('',(-12.973284400749,-26.5340597893858,8.9713386775021));
#96797=CARTESIAN_POINT('Origin',(-12.6801076948398,-26.5340598313603,8.90771935941597));
#96798=CARTESIAN_POINT('',(-13.06410080176,-25.9742356388815,8.52225303564387));
#96799=CARTESIAN_POINT('Origin',(-12.7692410021,-25.9742356128,8.46695657076));
#96800=CARTESIAN_POINT('Ctrl Pts',(-12.9732844032,-26.5340597894,8.9713386779));
#96801=CARTESIAN_POINT('Ctrl Pts',(-12.979891943676,-26.5239011923188,8.94088915075278));
#96802=CARTESIAN_POINT('Ctrl Pts',(-12.9862906228497,-26.5118121653252,
8.91097621606126));
#96803=CARTESIAN_POINT('Ctrl Pts',(-12.9924394245919,-26.4977670410124,
8.88184770694584));
#96804=CARTESIAN_POINT('Ctrl Pts',(-12.9980298766749,-26.4849973018402,
8.85536424865845));
#96805=CARTESIAN_POINT('Ctrl Pts',(-13.0034139204697,-26.4706087797295,
8.82952839709536));
#96806=CARTESIAN_POINT('Ctrl Pts',(-13.0085558742,-26.4545791221706,8.80456712582049));
#96807=CARTESIAN_POINT('Ctrl Pts',(-13.0131702409556,-26.4401941776882,
8.78216699031034));
#96808=CARTESIAN_POINT('Ctrl Pts',(-13.0175896851213,-26.4244868111922,
8.76047103867062));
#96809=CARTESIAN_POINT('Ctrl Pts',(-13.0217832115077,-26.4074544672131,
8.73968323166975));
#96810=CARTESIAN_POINT('Ctrl Pts',(-13.02367954228,-26.3997523675871,8.73028289541987));
#96811=CARTESIAN_POINT('Ctrl Pts',(-13.0255295972387,-26.3917795864622,
8.7210688510905));
#96812=CARTESIAN_POINT('Ctrl Pts',(-13.0273300783176,-26.383537525235,8.71206315735746));
#96813=CARTESIAN_POINT('Ctrl Pts',(-13.0306453306873,-26.3683612963176,
8.69548084064264));
#96814=CARTESIAN_POINT('Ctrl Pts',(-13.0337930017314,-26.3522696202503,
8.67960169725163));
#96815=CARTESIAN_POINT('Ctrl Pts',(-13.0367521637379,-26.3352719026803,
8.66456608725168));
#96816=CARTESIAN_POINT('Ctrl Pts',(-13.039820293027,-26.3176482663235,8.64897681051787));
#96817=CARTESIAN_POINT('Ctrl Pts',(-13.0426855701156,-26.299049974877,8.63429569933343));
#96818=CARTESIAN_POINT('Ctrl Pts',(-13.0453189403406,-26.2795297324795,
8.62071705815884));
#96819=CARTESIAN_POINT('Ctrl Pts',(-13.0479416652738,-26.2600883998665,
8.60719330808789));
#96820=CARTESIAN_POINT('Ctrl Pts',(-13.050334105218,-26.2397321641038,8.59476479434834));
#96821=CARTESIAN_POINT('Ctrl Pts',(-13.0524654801459,-26.2185617555089,
8.5836369832028));
#96822=CARTESIAN_POINT('Ctrl Pts',(-13.0544533237903,-26.1988170068846,
8.57325854233227));
#96823=CARTESIAN_POINT('Ctrl Pts',(-13.0562139011086,-26.178364235337,8.56401270697199));
#96824=CARTESIAN_POINT('Ctrl Pts',(-13.0577234588786,-26.157328093979,8.5560577868111));
#96825=CARTESIAN_POINT('Ctrl Pts',(-13.0591678057951,-26.1372006854713,
8.5484465084402));
#96826=CARTESIAN_POINT('Ctrl Pts',(-13.060382227609,-26.1165392613583,8.54201785128485));
#96827=CARTESIAN_POINT('Ctrl Pts',(-13.0613491801184,-26.0954923757779,
8.53688852111132));
#96828=CARTESIAN_POINT('Ctrl Pts',(-13.0622572570709,-26.0757269875808,
8.53207150428079));
#96829=CARTESIAN_POINT('Ctrl Pts',(-13.0629470166407,-26.0556218219351,
8.52840084562135));
#96830=CARTESIAN_POINT('Ctrl Pts',(-13.0634081609753,-26.0353336900326,
8.5259448160036));
#96831=CARTESIAN_POINT('Ctrl Pts',(-13.063868376796,-26.0150864082753,8.52349373160047));
#96832=CARTESIAN_POINT('Ctrl Pts',(-13.0641007978549,-25.9946567351865,
8.52225305135991));
#96833=CARTESIAN_POINT('Ctrl Pts',(-13.0641008048946,-25.9742356631,8.52225302771906));
#96834=CARTESIAN_POINT('Origin',(-12.7692410021,-27.9742356128,8.46695657076));
#96835=CARTESIAN_POINT('',(-13.0641007993,-27.8242356128,8.52225304435));
#96836=CARTESIAN_POINT('Origin',(2.84607155346,-26.5742356128,5.53854202767));
#96837=CARTESIAN_POINT('',(-3.40988736318,-26.5742356128,-9.39126352223));
#96838=CARTESIAN_POINT('Origin',(2.84607155346,-26.5742356128,5.53854202767));
#96839=CARTESIAN_POINT('Origin',(-3.29476681586543,-26.5721143161574,-9.11652914022926));
#96840=CARTESIAN_POINT('Ctrl Pts',(-3.40988736318,-26.5742356128,-9.39126352223));
#96841=CARTESIAN_POINT('Ctrl Pts',(-3.40988736318,-26.4799878332,-9.39126352223));
#96842=CARTESIAN_POINT('Ctrl Pts',(-3.39558379717,-26.3857400536,-9.35712815432));
#96843=CARTESIAN_POINT('Ctrl Pts',(-3.3667944876,-26.3112466293,-9.28842265298));
#96844=CARTESIAN_POINT('Ctrl Pts',(-3.33037075585,-26.2742356128,-9.20149765239));
#96845=CARTESIAN_POINT('Ctrl Pts',(-3.29394702409,-26.2742356128,-9.11457265181));
#96846=CARTESIAN_POINT('Ctrl Pts',(-3.4910113153,-26.5742356128,-9.3572705737));
#96847=CARTESIAN_POINT('Ctrl Pts',(-3.48037253295,-26.4769107573,-9.36172848744));
#96848=CARTESIAN_POINT('Ctrl Pts',(-3.45431071589,-26.3795859018,-9.32989979882));
#96849=CARTESIAN_POINT('Ctrl Pts',(-3.41483915768,-26.303996431,-9.26033984988));
#96850=CARTESIAN_POINT('Ctrl Pts',(-3.37184251989,-26.2694021533,-9.17077476858));
#96851=CARTESIAN_POINT('Ctrl Pts',(-3.33375727379,-26.2742356128,-9.08120968728));
#96852=CARTESIAN_POINT('Ctrl Pts',(-3.5717957464,-26.5610173226,-9.32277198251));
#96853=CARTESIAN_POINT('Ctrl Pts',(-3.54981186007,-26.4622981571,-9.33215415735));
#96854=CARTESIAN_POINT('Ctrl Pts',(-3.51119131997,-26.3635789917,-9.30295815815));
#96855=CARTESIAN_POINT('Ctrl Pts',(-3.46066295418,-26.2884340565,-9.23245787906));
#96856=CARTESIAN_POINT('Ctrl Pts',(-3.41172937916,-26.2574332304,-9.13990415856));
#96857=CARTESIAN_POINT('Ctrl Pts',(-3.37340074696,-26.2676265362,-9.04735043987));
#96858=CARTESIAN_POINT('Ctrl Pts',(-3.64994177161,-26.5349267151,-9.2887404003));
#96859=CARTESIAN_POINT('Ctrl Pts',(-3.61607413424,-26.4367209398,-9.30345845196));
#96860=CARTESIAN_POINT('Ctrl Pts',(-3.56428404035,-26.3385151645,-9.27721330878));
#96861=CARTESIAN_POINT('Ctrl Pts',(-3.50256972223,-26.2654317018,-9.20569945623));
#96862=CARTESIAN_POINT('Ctrl Pts',(-3.44864766071,-26.2389835875,-9.10982452003));
#96863=CARTESIAN_POINT('Ctrl Pts',(-3.41175001833,-26.2545810833,-9.01394958175));
#96864=CARTESIAN_POINT('Ctrl Pts',(-3.81424885473,-26.4476638797,-9.21588066878));
#96865=CARTESIAN_POINT('Ctrl Pts',(-3.75250256194,-26.3563393693,-9.24354676394));
#96866=CARTESIAN_POINT('Ctrl Pts',(-3.66984966637,-26.2650148589,-9.22480841607));
#96867=CARTESIAN_POINT('Ctrl Pts',(-3.58330407322,-26.2006837329,-9.15088080098));
#96868=CARTESIAN_POINT('Ctrl Pts',(-3.52146064047,-26.1853980321,-9.04666045675));
#96869=CARTESIAN_POINT('Ctrl Pts',(-3.4923805164,-26.2109498456,-8.94244011508));
#96870=CARTESIAN_POINT('Ctrl Pts',(-3.94071289979,-26.2993639395,-9.1578343834));
#96871=CARTESIAN_POINT('Ctrl Pts',(-3.85226553394,-26.2305560501,-9.19855372868));
#96872=CARTESIAN_POINT('Ctrl Pts',(-3.74014873645,-26.1617481608,-9.18796857302));
#96873=CARTESIAN_POINT('Ctrl Pts',(-3.63226461004,-26.1158647884,-9.11169933207));
#96874=CARTESIAN_POINT('Ctrl Pts',(-3.56907345668,-26.1106751416,-8.99858447989));
#96875=CARTESIAN_POINT('Ctrl Pts',(-3.55444130117,-26.1367996538,-8.88546962456));
#96876=CARTESIAN_POINT('Ctrl Pts',(-3.99426364762,-26.1995473566,-9.13275311113));
#96877=CARTESIAN_POINT('Ctrl Pts',(-3.89218061974,-26.1494194207,-9.18032667121));
#96878=CARTESIAN_POINT('Ctrl Pts',(-3.76509502836,-26.0992914848,-9.17426692037));
#96879=CARTESIAN_POINT('Ctrl Pts',(-3.64735025537,-26.0668944366,-9.09682188935));
#96880=CARTESIAN_POINT('Ctrl Pts',(-3.58578912303,-26.065499903,-8.97883752401));
#96881=CARTESIAN_POINT('Ctrl Pts',(-3.58072010307,-26.08689148,-8.86085315859));
#96882=CARTESIAN_POINT('Ctrl Pts',(-4.02121701032,-26.0867730682,-9.12012310673));
#96883=CARTESIAN_POINT('Ctrl Pts',(-3.9120664741,-26.0618073391,-9.17125792781));
#96884=CARTESIAN_POINT('Ctrl Pts',(-3.77723460736,-26.0368416101,-9.16757431204));
#96885=CARTESIAN_POINT('Ctrl Pts',(-3.65448289879,-26.0206759356,-9.08952658412));
#96886=CARTESIAN_POINT('Ctrl Pts',(-3.59394702701,-26.0199130168,-8.96899190369));
#96887=CARTESIAN_POINT('Ctrl Pts',(-3.59394702751,-26.0305043095,-8.84845722325));
#96888=CARTESIAN_POINT('Ctrl Pts',(-4.02121700383,-25.9742356142,-9.12012310922));
#96889=CARTESIAN_POINT('Ctrl Pts',(-3.91206646892,-25.9742356136,-9.17125793032));
#96890=CARTESIAN_POINT('Ctrl Pts',(-3.7772346035,-25.974235613,-9.16757431456));
#96891=CARTESIAN_POINT('Ctrl Pts',(-3.65448289578,-25.9742356126,-9.08952658662));
#96892=CARTESIAN_POINT('Ctrl Pts',(-3.59394702413,-25.9742356126,-8.96899190615));
#96893=CARTESIAN_POINT('Ctrl Pts',(-3.59394702414,-25.9742356128,-8.84845722568));
#96894=CARTESIAN_POINT('',(-4.02121700383,-25.9742356142,-9.12012310922));
#96895=CARTESIAN_POINT('Ctrl Pts',(-3.40988736318,-26.5742356128,-9.39126352223));
#96896=CARTESIAN_POINT('Ctrl Pts',(-3.4910113153,-26.5742356128,-9.3572705737));
#96897=CARTESIAN_POINT('Ctrl Pts',(-3.5717957464,-26.5610173226,-9.32277198251));
#96898=CARTESIAN_POINT('Ctrl Pts',(-3.64994177161,-26.5349267151,-9.2887404003));
#96899=CARTESIAN_POINT('Ctrl Pts',(-3.81424885473,-26.4476638797,-9.21588066878));
#96900=CARTESIAN_POINT('Ctrl Pts',(-3.94071289979,-26.2993639395,-9.1578343834));
#96901=CARTESIAN_POINT('Ctrl Pts',(-3.99426364762,-26.1995473566,-9.13275311113));
#96902=CARTESIAN_POINT('Ctrl Pts',(-4.02121701032,-26.0867730682,-9.12012310673));
#96903=CARTESIAN_POINT('Ctrl Pts',(-4.02121700383,-25.9742356142,-9.12012310922));
#96904=CARTESIAN_POINT('Ctrl Pts',(-3.59394702414,-25.9742356128,-8.84845722568));
#96905=CARTESIAN_POINT('Ctrl Pts',(-3.59394702413859,-25.9742356128,-8.86547082365358));
#96906=CARTESIAN_POINT('Ctrl Pts',(-3.59539869159477,-25.974235612795,-8.88248672119199));
#96907=CARTESIAN_POINT('Ctrl Pts',(-3.59828751216145,-25.9742356127898,
-8.89925093236573));
#96908=CARTESIAN_POINT('Ctrl Pts',(-3.60122870276565,-25.9742356127845,
-8.9163190538544));
#96909=CARTESIAN_POINT('Ctrl Pts',(-3.60565938344924,-25.9742356127791,
-8.93312594622168));
#96910=CARTESIAN_POINT('Ctrl Pts',(-3.61151215671489,-25.9742356127769,
-8.94941892221616));
#96911=CARTESIAN_POINT('Ctrl Pts',(-3.61752207494251,-25.9742356127746,
-8.9661493590479));
#96912=CARTESIAN_POINT('Ctrl Pts',(-3.62503123537727,-25.9742356127756,
-8.98233749575522));
#96913=CARTESIAN_POINT('Ctrl Pts',(-3.63391585030532,-25.9742356127818,
-8.99773161493334));
#96914=CARTESIAN_POINT('Ctrl Pts',(-3.64291284694615,-25.9742356127882,
-9.01332045470364));
#96915=CARTESIAN_POINT('Ctrl Pts',(-3.65331989483763,-25.9742356127999,
-9.02809466264263));
#96916=CARTESIAN_POINT('Ctrl Pts',(-3.66496225633728,-25.9742356128182,
-9.04182116714993));
#96917=CARTESIAN_POINT('Ctrl Pts',(-3.67676344198006,-25.9742356128368,
-9.05573492750878));
#96918=CARTESIAN_POINT('Ctrl Pts',(-3.68983340448778,-25.9742356128621,
-9.06857177135196));
#96919=CARTESIAN_POINT('Ctrl Pts',(-3.70394976533629,-25.9742356128952,
-9.08012422995346));
#96920=CARTESIAN_POINT('Ctrl Pts',(-3.71326866162606,-25.9742356129171,
-9.08775056968468));
#96921=CARTESIAN_POINT('Ctrl Pts',(-3.72304275512652,-25.9742356129423,
-9.09481791747569));
#96922=CARTESIAN_POINT('Ctrl Pts',(-3.73320020269621,-25.9742356129715,
-9.10127620403795));
#96923=CARTESIAN_POINT('Ctrl Pts',(-3.74860166909693,-25.9742356130157,
-9.11106873142366));
#96924=CARTESIAN_POINT('Ctrl Pts',(-3.76489842790395,-25.9742356130674,
-9.11946694152528));
#96925=CARTESIAN_POINT('Ctrl Pts',(-3.78182194867813,-25.9742356131258,
-9.12632585130464));
#96926=CARTESIAN_POINT('Ctrl Pts',(-3.79860151107297,-25.9742356131837,
-9.1331264163962));
#96927=CARTESIAN_POINT('Ctrl Pts',(-3.81599663952131,-25.9742356132481,
-9.13841346048746));
#96928=CARTESIAN_POINT('Ctrl Pts',(-3.83372562740725,-25.9742356133179,
-9.1420926721867));
#96929=CARTESIAN_POINT('Ctrl Pts',(-3.85107739541277,-25.9742356133862,
-9.14569360125604));
#96930=CARTESIAN_POINT('Ctrl Pts',(-3.86874841653982,-25.9742356134597,
-9.14775424225408));
#96931=CARTESIAN_POINT('Ctrl Pts',(-3.88646372344271,-25.9742356135371,
-9.14823449310598));
#96932=CARTESIAN_POINT('Ctrl Pts',(-3.90391680093427,-25.9742356136134,
-9.14870763508312));
#96933=CARTESIAN_POINT('Ctrl Pts',(-3.92141238189434,-25.9742356136936,
-9.14764666810675));
#96934=CARTESIAN_POINT('Ctrl Pts',(-3.93868441830445,-25.9742356137763,
-9.145062978613));
#96935=CARTESIAN_POINT('Ctrl Pts',(-3.95554177681329,-25.9742356138571,
-9.14254131995981));
#96936=CARTESIAN_POINT('Ctrl Pts',(-3.97218578514195,-25.9742356139402,
-9.13856913641943));
#96937=CARTESIAN_POINT('Ctrl Pts',(-3.98837262606647,-25.9742356140244,
-9.1332060827271));
#96938=CARTESIAN_POINT('Ctrl Pts',(-3.99956528614096,-25.9742356140826,
-9.12949771015339));
#96939=CARTESIAN_POINT('Ctrl Pts',(-4.0105394337227,-25.9742356141413,-9.12512533516117));
#96940=CARTESIAN_POINT('Ctrl Pts',(-4.02121700383,-25.9742356142,-9.12012310922));
#96941=CARTESIAN_POINT('Origin',(-3.89394702409,-27.9742356128,-8.84845722572));
#96942=CARTESIAN_POINT('',(-4.02121700373,-27.8242356128,-9.12012310927));
#96943=CARTESIAN_POINT('Origin',(2.84607155346,-27.8242356128,5.53854202767));
#96944=CARTESIAN_POINT('',(-12.9732844032,-27.8242356128,8.9713386779));
#96945=CARTESIAN_POINT('Origin',(10.0415172382,-26.5742356128,8.33514586886));
#96946=CARTESIAN_POINT('',(12.9037784987484,-26.5742355987284,9.23373391245544));
#96947=CARTESIAN_POINT('Origin',(12.6175523690299,-26.5742356128,9.14387512190451));
#96948=CARTESIAN_POINT('',(12.4158605957,-26.5742356128,10.1688562115));
#96949=CARTESIAN_POINT('Origin',(12.1784262599,-26.5742356128,9.98548517727));
#96950=CARTESIAN_POINT('Origin',(10.0415172382,-26.5742356128,8.33514586886));
#96951=CARTESIAN_POINT('Ctrl Pts',(12.6068339386,-26.2541477285,8.98696689141));
#96952=CARTESIAN_POINT('Ctrl Pts',(12.7066930633,-26.2358983992,9.01483962091));
#96953=CARTESIAN_POINT('Ctrl Pts',(12.8178300069,-26.2607313227,9.03051509132));
#96954=CARTESIAN_POINT('Ctrl Pts',(12.9140852431,-26.3342556033,9.02641004159));
#96955=CARTESIAN_POINT('Ctrl Pts',(12.9662467501,-26.4341577237,9.00377029278));
#96956=CARTESIAN_POINT('Ctrl Pts',(12.9732844032,-26.5340598441,8.9713386779));
#96957=CARTESIAN_POINT('Ctrl Pts',(12.6106280003,-26.2619885586,9.01816975155));
#96958=CARTESIAN_POINT('Ctrl Pts',(12.708974138,-26.2477664531,9.04491835482));
#96959=CARTESIAN_POINT('Ctrl Pts',(12.8159524428,-26.2758436136,9.06233104132));
#96960=CARTESIAN_POINT('Ctrl Pts',(12.9070210129,-26.3504586067,9.06354827381));
#96961=CARTESIAN_POINT('Ctrl Pts',(12.9560253652,-26.4501000555,9.04813737607));
#96962=CARTESIAN_POINT('Ctrl Pts',(12.9621611611,-26.5497415044,9.02259791155));
#96963=CARTESIAN_POINT('Ctrl Pts',(12.6136807588,-26.2679937272,9.04969534782));
#96964=CARTESIAN_POINT('Ctrl Pts',(12.7102354837,-26.2577528513,9.0760062137));
#96965=CARTESIAN_POINT('Ctrl Pts',(12.8129790795,-26.2887376058,9.09562365218));
#96966=CARTESIAN_POINT('Ctrl Pts',(12.8989313579,-26.3639769508,9.10215295496));
#96967=CARTESIAN_POINT('Ctrl Pts',(12.9446683244,-26.4628643491,9.09369562263));
#96968=CARTESIAN_POINT('Ctrl Pts',(12.949656063,-26.5617517538,9.07481948836));
#96969=CARTESIAN_POINT('Ctrl Pts',(12.6158914118,-26.2721121063,9.08130970942));
#96970=CARTESIAN_POINT('Ctrl Pts',(12.7104096761,-26.2656378329,9.10778259443));
#96971=CARTESIAN_POINT('Ctrl Pts',(12.8088747795,-26.2991108653,9.12998686861));
#96972=CARTESIAN_POINT('Ctrl Pts',(12.8897865248,-26.3745377171,9.1418082035));
#96973=CARTESIAN_POINT('Ctrl Pts',(12.9321497434,-26.4722631499,9.14006801201));
#96974=CARTESIAN_POINT('Ctrl Pts',(12.9357345368,-26.5699885837,9.12765954366));
#96975=CARTESIAN_POINT('Ctrl Pts',(12.6171883094,-26.2742355975,9.11279216515));
#96976=CARTESIAN_POINT('Ctrl Pts',(12.7094740156,-26.2712015816,9.13993707984));
#96977=CARTESIAN_POINT('Ctrl Pts',(12.8036505085,-26.3066955811,9.16503705887));
#96978=CARTESIAN_POINT('Ctrl Pts',(12.8795985938,-26.3818769922,9.18212527582));
#96979=CARTESIAN_POINT('Ctrl Pts',(12.9184829148,-26.4780562725,9.18689609473));
#96980=CARTESIAN_POINT('Ctrl Pts',(12.9204030457,-26.5742355538,9.18077993753));
#96981=CARTESIAN_POINT('Ctrl Pts',(12.6175523411,-26.2742356062,9.14387513829));
#96982=CARTESIAN_POINT('Ctrl Pts',(12.7074729361,-26.2742356042,9.17210511002));
#96983=CARTESIAN_POINT('Ctrl Pts',(12.7973935329,-26.311246617,9.20033507989));
#96984=CARTESIAN_POINT('Ctrl Pts',(12.8684667546,-26.3857400362,9.22264803953));
#96985=CARTESIAN_POINT('Ctrl Pts',(12.9037784934,-26.4799878104,9.23373391858));
#96986=CARTESIAN_POINT('Ctrl Pts',(12.9037784969,-26.574235585,9.23373391359));
#96987=CARTESIAN_POINT('Ctrl Pts',(12.9732843928317,-26.5340598587174,8.97133872568045));
#96988=CARTESIAN_POINT('Ctrl Pts',(12.9674428625711,-26.54229530553,8.99825824592988));
#96989=CARTESIAN_POINT('Ctrl Pts',(12.9612109795608,-26.5492260544689,9.02518736608815));
#96990=CARTESIAN_POINT('Ctrl Pts',(12.9545858707363,-26.5549069523633,9.05210598814747));
#96991=CARTESIAN_POINT('Ctrl Pts',(12.9478040477681,-26.5607222294918,9.07966135881259));
#96992=CARTESIAN_POINT('Ctrl Pts',(12.9406099943118,-26.5652277143943,9.10720670287461));
#96993=CARTESIAN_POINT('Ctrl Pts',(12.9329983321515,-26.5684286387089,9.13473197822653));
#96994=CARTESIAN_POINT('Ctrl Pts',(12.9254138081857,-26.571618150627,9.16215911650105));
#96995=CARTESIAN_POINT('Ctrl Pts',(12.9174143717085,-26.5735122847671,9.18956733401115));
#96996=CARTESIAN_POINT('Ctrl Pts',(12.9089958566211,-26.574065542159,9.21694310775132));
#96997=CARTESIAN_POINT('Ctrl Pts',(12.9072742542534,-26.5741786843492,9.22254150561577));
#96998=CARTESIAN_POINT('Ctrl Pts',(12.905535138156,-26.5742355816927,9.22813850523854));
#96999=CARTESIAN_POINT('Ctrl Pts',(12.9037784973901,-26.574235585,9.23373391202899));
#97000=CARTESIAN_POINT('Origin',(10.0415172382,-27.8242356128,8.33514586886));
#97001=CARTESIAN_POINT('',(12.4158605957,-27.8242356128,10.1688562115));
#97002=CARTESIAN_POINT('Origin',(-10.0415172382,-26.5742356128,8.33514586886));
#97003=CARTESIAN_POINT('',(-12.4158605957,-26.5742356128,10.1688562115));
#97004=CARTESIAN_POINT('Origin',(-12.1784262599,-26.5742356128,9.98548517727));
#97005=CARTESIAN_POINT('',(-12.9037784845,-26.5742356128,9.23373396017));
#97006=CARTESIAN_POINT('Origin',(-12.6195762561711,-26.5721143167766,9.14451056062222));
#97007=CARTESIAN_POINT('Origin',(-10.0415172382,-26.5742356128,8.33514586886));
#97008=CARTESIAN_POINT('Ctrl Pts',(-12.6175523599,-26.2742356128,9.14387515104));
#97009=CARTESIAN_POINT('Ctrl Pts',(-12.7074729489,-26.2742356128,9.1721051285));
#97010=CARTESIAN_POINT('Ctrl Pts',(-12.7973935379,-26.3112466293,9.20033510596));
#97011=CARTESIAN_POINT('Ctrl Pts',(-12.8684667518,-26.3857400536,9.22264807394));
#97012=CARTESIAN_POINT('Ctrl Pts',(-12.9037784845,-26.4799878332,9.23373396017));
#97013=CARTESIAN_POINT('Ctrl Pts',(-12.9037784845,-26.5742356128,9.23373396017));
#97014=CARTESIAN_POINT('Ctrl Pts',(-12.6171883574,-26.2742356128,9.11279315844));
#97015=CARTESIAN_POINT('Ctrl Pts',(-12.7094739788,-26.2712016953,9.13993811731));
#97016=CARTESIAN_POINT('Ctrl Pts',(-12.8036503248,-26.3066957496,9.1650382076));
#97017=CARTESIAN_POINT('Ctrl Pts',(-12.8795982434,-26.3818771498,9.18212660258));
#97018=CARTESIAN_POINT('Ctrl Pts',(-12.9184824419,-26.4780563813,9.18689763116));
#97019=CARTESIAN_POINT('Ctrl Pts',(-12.9204025066,-26.5742356128,9.18078167336));
#97020=CARTESIAN_POINT('Ctrl Pts',(-12.6158916105,-26.2721122483,9.0813123221));
#97021=CARTESIAN_POINT('Ctrl Pts',(-12.7104096521,-26.2656382627,9.10778530133));
#97022=CARTESIAN_POINT('Ctrl Pts',(-12.8088743595,-26.2991114721,9.12998985719));
#97023=CARTESIAN_POINT('Ctrl Pts',(-12.8897856562,-26.3745383201,9.14181166467));
#97024=CARTESIAN_POINT('Ctrl Pts',(-12.9321485573,-26.4722636434,9.1400720384));
#97025=CARTESIAN_POINT('Ctrl Pts',(-12.9357331951,-26.5699889642,9.12766410551));
#97026=CARTESIAN_POINT('Ctrl Pts',(-12.6136812731,-26.2679944507,9.04969907596));
#97027=CARTESIAN_POINT('Ctrl Pts',(-12.7102357572,-26.257754074,9.07600987399));
#97028=CARTESIAN_POINT('Ctrl Pts',(-12.8129788034,-26.28873921,9.09562757859));
#97029=CARTESIAN_POINT('Ctrl Pts',(-12.8989304246,-26.363978659,9.10215754682));
#97030=CARTESIAN_POINT('Ctrl Pts',(-12.944666986,-26.4628659856,9.09370108211));
#97031=CARTESIAN_POINT('Ctrl Pts',(-12.9496546007,-26.5617533112,9.074825766));
#97032=CARTESIAN_POINT('Ctrl Pts',(-12.6106281314,-26.26198871,9.01817066751));
#97033=CARTESIAN_POINT('Ctrl Pts',(-12.708974212,-26.2477667318,9.04491924544));
#97034=CARTESIAN_POINT('Ctrl Pts',(-12.8159523793,-26.2758439872,9.06233199343));
#97035=CARTESIAN_POINT('Ctrl Pts',(-12.9070207823,-26.350459,9.06354939385));
#97036=CARTESIAN_POINT('Ctrl Pts',(-12.9560250323,-26.4501004207,9.04813871743));
#97037=CARTESIAN_POINT('Ctrl Pts',(-12.9621607982,-26.5497418392,9.02259946049));
#97038=CARTESIAN_POINT('Ctrl Pts',(-12.6068339484,-26.2541476936,8.98696687838));
#97039=CARTESIAN_POINT('Ctrl Pts',(-12.7066930674,-26.2358983672,9.01483961189));
#97040=CARTESIAN_POINT('Ctrl Pts',(-12.8178300052,-26.2607312902,9.0305150864));
#97041=CARTESIAN_POINT('Ctrl Pts',(-12.9140852366,-26.3342555659,9.02641003965));
#97042=CARTESIAN_POINT('Ctrl Pts',(-12.9662467409,-26.4341576782,9.00377029183));
#97043=CARTESIAN_POINT('Ctrl Pts',(-12.9732843934,-26.5340597894,8.97133867629));
#97044=CARTESIAN_POINT('Ctrl Pts',(-12.9037784845,-26.5742356128,9.23373396017));
#97045=CARTESIAN_POINT('Ctrl Pts',(-12.9123899316053,-26.5742356128,9.20630402689466));
#97046=CARTESIAN_POINT('Ctrl Pts',(-12.9205796598355,-26.5728724678115,
9.17883767519317));
#97047=CARTESIAN_POINT('Ctrl Pts',(-12.9283513177015,-26.5702022988638,
9.15135033698744));
#97048=CARTESIAN_POINT('Ctrl Pts',(-12.9361496963363,-26.5675229492537,
9.1237684909151));
#97049=CARTESIAN_POINT('Ctrl Pts',(-12.9435274399562,-26.5635275942613,
9.09616440770698));
#97050=CARTESIAN_POINT('Ctrl Pts',(-12.9504901127122,-26.5582212495112,
9.06854732983508));
#97051=CARTESIAN_POINT('Ctrl Pts',(-12.9572170081428,-26.5530945937709,
9.04186545041132));
#97052=CARTESIAN_POINT('Ctrl Pts',(-12.9635566560319,-26.5467441560851,
9.01517048220121));
#97053=CARTESIAN_POINT('Ctrl Pts',(-12.9695122335975,-26.5391272012899,
8.9884798091082));
#97054=CARTESIAN_POINT('Ctrl Pts',(-12.9707872326892,-26.537496526458,8.98276573963696));
#97055=CARTESIAN_POINT('Ctrl Pts',(-12.9720446165679,-26.5358076273671,
8.97705193099787));
#97056=CARTESIAN_POINT('Ctrl Pts',(-12.9732843934,-26.5340597894,8.97133867629));
#97057=CARTESIAN_POINT('Origin',(-10.0415172382,-27.8242356128,8.33514586886));
#97058=CARTESIAN_POINT('',(-12.4158605957,-27.8242356128,10.1688562115));
#97059=CARTESIAN_POINT('Origin',(-8.72866611926,-23.4742356128,13.252332246));
#97060=CARTESIAN_POINT('',(-8.89884287263,-23.4742356128,13.4993947332));
#97061=CARTESIAN_POINT('Origin',(-8.72866611926,-23.4742356128,13.252332246));
#97062=CARTESIAN_POINT('Origin',(-8.72866611926,-23.4742356128,13.252332246));
#97063=CARTESIAN_POINT('',(-8.78700378468238,-23.1849482466887,13.3062723665177));
#97064=CARTESIAN_POINT('Origin',(-8.72866611926,-23.4742356128,13.252332246));
#97065=CARTESIAN_POINT('Origin',(8.72866611926,-23.4742356128,13.252332246));
#97066=CARTESIAN_POINT('',(8.89884287263,-23.4742356128,13.4993947332));
#97067=CARTESIAN_POINT('',(8.94893776852305,-23.4742356128,13.4559996231887));
#97068=CARTESIAN_POINT('Origin',(8.72866611926,-23.4742356128,13.252332246));
#97069=CARTESIAN_POINT('',(8.94177659881935,-23.3983621101791,13.4493782688019));
#97070=CARTESIAN_POINT('Origin',(8.72866611926,-23.4742356128,13.252332246));
#97071=CARTESIAN_POINT('Origin',(8.72866611926,-23.4742356128,13.252332246));
#97072=CARTESIAN_POINT('Origin',(8.72866611926,-23.4742356128,13.252332246));
#97073=CARTESIAN_POINT('Origin',(5.43994370138E-15,-23.4742356128,0.580061096523));
#97074=CARTESIAN_POINT('Origin',(1.10873183178E-16,-23.4742356128,0.580061096523));
#97075=CARTESIAN_POINT('Origin',(-2.04512416396E-15,-26.5742356128,0.580061096523));
#97076=CARTESIAN_POINT('',(-9.40585242867367,-26.5742358357554,13.1350810502009));
#97077=CARTESIAN_POINT('Origin',(-9.22597996127761,-26.5742356128,12.8949854593485));
#97078=CARTESIAN_POINT('Origin',(-2.68767324558E-16,-26.5742356128,0.580061096523));
#97079=CARTESIAN_POINT('Ctrl Pts',(-8.93233349645,-25.9742356128,13.0320605967));
#97080=CARTESIAN_POINT('Ctrl Pts',(-9.0112864001,-25.9742356128,13.1050619605));
#97081=CARTESIAN_POINT('Ctrl Pts',(-9.05753156728,-25.9742356128,13.2134376055));
#97082=CARTESIAN_POINT('Ctrl Pts',(-9.04862484094,-25.9742356128,13.3377236529));
#97083=CARTESIAN_POINT('Ctrl Pts',(-8.98739853023,-25.9742356128,13.4383975561));
#97084=CARTESIAN_POINT('Ctrl Pts',(-8.89884287263,-25.9742356128,13.4993947332));
#97085=CARTESIAN_POINT('Ctrl Pts',(-8.93233349645,-26.0285372111,13.0320605967));
#97086=CARTESIAN_POINT('Ctrl Pts',(-9.0112864001,-26.0241566749,13.1050619605));
#97087=CARTESIAN_POINT('Ctrl Pts',(-9.05753156726,-26.0284966165,13.2134376055));
#97088=CARTESIAN_POINT('Ctrl Pts',(-9.04862484095,-26.0429379832,13.3377236529));
#97089=CARTESIAN_POINT('Ctrl Pts',(-8.98739853023,-26.0628883963,13.4383975561));
#97090=CARTESIAN_POINT('Ctrl Pts',(-8.89884287263,-26.0828388094,13.4993947332));
#97091=CARTESIAN_POINT('Ctrl Pts',(-8.94472655074,-26.08285904,13.0267961436));
#97092=CARTESIAN_POINT('Ctrl Pts',(-9.02169065378,-26.074050391,13.1006602186));
#97093=CARTESIAN_POINT('Ctrl Pts',(-9.06768131823,-26.0827027622,13.2080228858));
#97094=CARTESIAN_POINT('Ctrl Pts',(-9.06113122668,-26.1115995645,13.3293879943));
#97095=CARTESIAN_POINT('Ctrl Pts',(-9.00408533535,-26.1515406257,13.4266880848));
#97096=CARTESIAN_POINT('Ctrl Pts',(-8.91997599276,-26.1914817452,13.4848363629));
#97097=CARTESIAN_POINT('Ctrl Pts',(-8.9695742685,-26.1326166293,13.016255239));
#97098=CARTESIAN_POINT('Ctrl Pts',(-9.04255123506,-26.1212616413,13.0918512663));
#97099=CARTESIAN_POINT('Ctrl Pts',(-9.08803799129,-26.134748461,13.1971786824));
#97100=CARTESIAN_POINT('Ctrl Pts',(-9.08621282797,-26.1765733467,13.3126866711));
#97101=CARTESIAN_POINT('Ctrl Pts',(-9.03754117443,-26.2337854443,13.4032271249));
#97102=CARTESIAN_POINT('Ctrl Pts',(-8.96233987903,-26.290997548,13.4556696979));
#97103=CARTESIAN_POINT('Ctrl Pts',(-9.03028791925,-26.2079395652,12.989613417));
#97104=CARTESIAN_POINT('Ctrl Pts',(-9.09589435053,-26.1961913738,13.0677079223));
#97105=CARTESIAN_POINT('Ctrl Pts',(-9.14175144084,-26.2188939721,13.1671618616));
#97106=CARTESIAN_POINT('Ctrl Pts',(-9.15122220031,-26.2795381045,13.2688142601));
#97107=CARTESIAN_POINT('Ctrl Pts',(-9.12142423198,-26.3605908527,13.3437756344));
#97108=CARTESIAN_POINT('Ctrl Pts',(-9.06630530821,-26.4416435958,13.3830106592));
#97109=CARTESIAN_POINT('Ctrl Pts',(-9.1104960852,-26.2536276545,12.9522433826));
#97110=CARTESIAN_POINT('Ctrl Pts',(-9.1703946836,-26.2462276286,13.0306868925));
#97111=CARTESIAN_POINT('Ctrl Pts',(-9.21936149245,-26.2769167679,13.1209534215));
#97112=CARTESIAN_POINT('Ctrl Pts',(-9.24339400518,-26.3479556515,13.2050413138));
#97113=CARTESIAN_POINT('Ctrl Pts',(-9.23603570877,-26.4404876405,13.260825769));
#97114=CARTESIAN_POINT('Ctrl Pts',(-9.20475552832,-26.5330196335,13.28361302));
#97115=CARTESIAN_POINT('Ctrl Pts',(-9.14847854779,-26.2673388385,12.9340159562));
#97116=CARTESIAN_POINT('Ctrl Pts',(-9.2065559864,-26.2624721802,13.0119783221));
#97117=CARTESIAN_POINT('Ctrl Pts',(-9.2575613966,-26.2961769579,13.0975892735));
#97118=CARTESIAN_POINT('Ctrl Pts',(-9.28841654251,-26.3700572474,13.1735175604));
#97119=CARTESIAN_POINT('Ctrl Pts',(-9.29115586865,-26.4652497721,13.2205120876));
#97120=CARTESIAN_POINT('Ctrl Pts',(-9.27058953184,-26.5604422808,13.2357088969));
#97121=CARTESIAN_POINT('Ctrl Pts',(-9.18739830238,-26.274235893,12.9147116237));
#97122=CARTESIAN_POINT('Ctrl Pts',(-9.24438226141,-26.2719282776,12.9916193734));
#97123=CARTESIAN_POINT('Ctrl Pts',(-9.2979593505,-26.307785511,13.072211743));
#97124=CARTESIAN_POINT('Ctrl Pts',(-9.33575986597,-26.382802277,13.1399052833));
#97125=CARTESIAN_POINT('Ctrl Pts',(-9.34842419719,-26.4785192081,13.1781045816));
#97126=CARTESIAN_POINT('Ctrl Pts',(-9.33836508495,-26.5742361412,13.1856405721));
#97127=CARTESIAN_POINT('Ctrl Pts',(-9.22598003346,-26.2742358377,12.8949853402));
#97128=CARTESIAN_POINT('Ctrl Pts',(-9.28248863171,-26.2742358325,12.9704136123));
#97129=CARTESIAN_POINT('Ctrl Pts',(-9.33899722271,-26.3112468736,13.0458418922));
#97130=CARTESIAN_POINT('Ctrl Pts',(-9.38366159094,-26.3857403537,13.1054603965));
#97131=CARTESIAN_POINT('Ctrl Pts',(-9.40585244492,-26.4799882059,13.1350810267));
#97132=CARTESIAN_POINT('Ctrl Pts',(-9.40585242353,-26.5742360581,13.1350810427));
#97133=CARTESIAN_POINT('',(-8.89884287263,-25.9742356128,13.4993947332));
#97134=CARTESIAN_POINT('Ctrl Pts',(-8.89884287263,-25.9742356128,13.4993947332));
#97135=CARTESIAN_POINT('Ctrl Pts',(-8.98739853023,-25.9742356128002,13.4383975561));
#97136=CARTESIAN_POINT('Ctrl Pts',(-9.04862484094,-25.9742356128001,13.3377236529));
#97137=CARTESIAN_POINT('Ctrl Pts',(-9.05753156728,-25.9742356128001,13.2134376055));
#97138=CARTESIAN_POINT('Ctrl Pts',(-9.0112864001,-25.9742356128001,13.1050619605));
#97139=CARTESIAN_POINT('Ctrl Pts',(-8.93233349645,-25.9742356128,13.0320605967));
#97140=CARTESIAN_POINT('Ctrl Pts',(-8.89884287263,-25.9742356128,13.4993947332));
#97141=CARTESIAN_POINT('Ctrl Pts',(-8.89895609808286,-26.0010432829593,
13.4993167434567));
#97142=CARTESIAN_POINT('Ctrl Pts',(-8.90059919950406,-26.0277666642535,
13.4981851695452));
#97143=CARTESIAN_POINT('Ctrl Pts',(-8.90372878865397,-26.0541518085826,
13.496027640683));
#97144=CARTESIAN_POINT('Ctrl Pts',(-8.90702142789706,-26.081911606272,13.4937577056022));
#97145=CARTESIAN_POINT('Ctrl Pts',(-8.91195898935124,-26.1092969617299,
13.4903524012086));
#97146=CARTESIAN_POINT('Ctrl Pts',(-8.91844967243714,-26.1360470459536,
13.4858669737749));
#97147=CARTESIAN_POINT('Ctrl Pts',(-8.92544355331223,-26.1648709617083,
13.4810338083391));
#97148=CARTESIAN_POINT('Ctrl Pts',(-8.93424021215507,-26.1929569983882,
13.4749468232508));
#97149=CARTESIAN_POINT('Ctrl Pts',(-8.94468577595512,-26.2200211365478,
13.4676969887184));
#97150=CARTESIAN_POINT('Ctrl Pts',(-8.95549613608157,-26.2480304508958,
13.4601939641185));
#97151=CARTESIAN_POINT('Ctrl Pts',(-8.96807170222389,-26.2749450857715,
13.451445930878));
#97152=CARTESIAN_POINT('Ctrl Pts',(-8.98221286723584,-26.3004968966248,
13.4415701314541));
#97153=CARTESIAN_POINT('Ctrl Pts',(-8.99656295183038,-26.3264262063373,
13.4315484283587));
#97154=CARTESIAN_POINT('Ctrl Pts',(-9.01252419020305,-26.3509519159204,
13.4203659558918));
#97155=CARTESIAN_POINT('Ctrl Pts',(-9.02987348408223,-26.3738436039025,
13.4081537502609));
#97156=CARTESIAN_POINT('Ctrl Pts',(-9.03813067124657,-26.3847386266909,
13.4023414982877));
#97157=CARTESIAN_POINT('Ctrl Pts',(-9.04670216437771,-26.3952642555391,
13.3962960646772));
#97158=CARTESIAN_POINT('Ctrl Pts',(-9.05556386016477,-26.4053998182991,
13.3900316588417));
#97159=CARTESIAN_POINT('Ctrl Pts',(-9.06617082519398,-26.417531532401,13.3825335077853));
#97160=CARTESIAN_POINT('Ctrl Pts',(-9.07717152666241,-26.4290529763397,
13.3747371662871));
#97161=CARTESIAN_POINT('Ctrl Pts',(-9.08851925551041,-26.4399493747432,
13.3666713990996));
#97162=CARTESIAN_POINT('Ctrl Pts',(-9.10945377975007,-26.4600512752697,
13.3517915054257));
#97163=CARTESIAN_POINT('Ctrl Pts',(-9.13156720191249,-26.4780257582573,
13.3359958573705));
#97164=CARTESIAN_POINT('Ctrl Pts',(-9.1545917526907,-26.493783803096,13.319450281518));
#97165=CARTESIAN_POINT('Ctrl Pts',(-9.17536032095728,-26.5079978493604,
13.3045258677949));
#97166=CARTESIAN_POINT('Ctrl Pts',(-9.19687135475279,-26.520409644557,13.2889905507415));
#97167=CARTESIAN_POINT('Ctrl Pts',(-9.21895271273267,-26.5309615712851,
13.2729526717885));
#97168=CARTESIAN_POINT('Ctrl Pts',(-9.2368976785699,-26.5395368574983,13.2599190897881));
#97169=CARTESIAN_POINT('Ctrl Pts',(-9.25507229474382,-26.5468177853716,
13.2466605914074));
#97170=CARTESIAN_POINT('Ctrl Pts',(-9.27346468079951,-26.5528426061672,
13.2331808449775));
#97171=CARTESIAN_POINT('Ctrl Pts',(-9.29181826304442,-26.5588547159418,
13.2197295377903));
#97172=CARTESIAN_POINT('Ctrl Pts',(-9.31038957007988,-26.5636163178449,
13.2060573013725));
#97173=CARTESIAN_POINT('Ctrl Pts',(-9.32918002295672,-26.5671165247323,
13.1921579856977));
#97174=CARTESIAN_POINT('Ctrl Pts',(-9.34748417167067,-26.5705261449163,
13.1786183896698));
#97175=CARTESIAN_POINT('Ctrl Pts',(-9.36599704153926,-26.5727388942514,
13.1648627383229));
#97176=CARTESIAN_POINT('Ctrl Pts',(-9.38472045559965,-26.5736958247132,
13.1508847837228));
#97177=CARTESIAN_POINT('Ctrl Pts',(-9.39173501954148,-26.5740543303731,
13.1456480648209));
#97178=CARTESIAN_POINT('Ctrl Pts',(-9.39877908188713,-26.5742360668045,
13.1403801822461));
#97179=CARTESIAN_POINT('Ctrl Pts',(-9.40585242322525,-26.5742360581,13.1350810429283));
#97180=CARTESIAN_POINT('Origin',(-8.72866611926,-27.9742356128,13.252332246));
#97181=CARTESIAN_POINT('',(-8.89884287263,-27.8242356128,13.4993947332));
#97182=CARTESIAN_POINT('Origin',(1.50758951484E-15,-26.5742356128,0.580061096523));
#97183=CARTESIAN_POINT('',(9.40585256108342,-26.5742356128,13.1350809262965));
#97184=CARTESIAN_POINT('Origin',(9.22725087823104,-26.5721145657866,12.8966831494532));
#97185=CARTESIAN_POINT('Origin',(-2.68767324558E-16,-26.5742356128,0.580061096523));
#97186=CARTESIAN_POINT('Ctrl Pts',(9.22598017922,-26.2742358667,12.8949853208));
#97187=CARTESIAN_POINT('Ctrl Pts',(9.28248884108,-26.2742358731,12.9704135146));
#97188=CARTESIAN_POINT('Ctrl Pts',(9.33899753074,-26.3112469248,13.0458416783));
#97189=CARTESIAN_POINT('Ctrl Pts',(9.38366202162,-26.385740412,13.105460047));
#97190=CARTESIAN_POINT('Ctrl Pts',(9.40585299479,-26.4799882688,13.1350805566));
#97191=CARTESIAN_POINT('Ctrl Pts',(9.40585306927,-26.5742361254,13.1350804849));
#97192=CARTESIAN_POINT('Ctrl Pts',(9.18809325963,-26.2742357357,12.9143563956));
#97193=CARTESIAN_POINT('Ctrl Pts',(9.2450687066,-26.2719697063,12.9912374316));
#97194=CARTESIAN_POINT('Ctrl Pts',(9.29869866779,-26.3078477237,13.071736699));
#97195=CARTESIAN_POINT('Ctrl Pts',(9.3366228955,-26.3828550411,13.1392846998));
#97196=CARTESIAN_POINT('Ctrl Pts',(9.34945889077,-26.478545471,13.1773294073));
#97197=CARTESIAN_POINT('Ctrl Pts',(9.33958101525,-26.5742358983,13.1847296173));
#97198=CARTESIAN_POINT('Ctrl Pts',(9.14988050464,-26.2675847856,12.9333199946));
#97199=CARTESIAN_POINT('Ctrl Pts',(9.20791871134,-26.2628099114,13.0112443559));
#97200=CARTESIAN_POINT('Ctrl Pts',(9.25901673093,-26.2965916112,13.096674713));
#97201=CARTESIAN_POINT('Ctrl Pts',(9.29012180691,-26.3705121727,13.1723066998));
#97202=CARTESIAN_POINT('Ctrl Pts',(9.29321828466,-26.4657229441,13.218984685));
#97203=CARTESIAN_POINT('Ctrl Pts',(9.2730301115,-26.5609337322,13.2339056769));
#97204=CARTESIAN_POINT('Ctrl Pts',(9.112555303,-26.2543622577,12.9512548511));
#97205=CARTESIAN_POINT('Ctrl Pts',(9.17235549832,-26.2470995345,13.0296719809));
#97206=CARTESIAN_POINT('Ctrl Pts',(9.22143309124,-26.2779511011,13.1196858885));
#97207=CARTESIAN_POINT('Ctrl Pts',(9.24583568971,-26.3491419477,13.2033312194));
#97208=CARTESIAN_POINT('Ctrl Pts',(9.23902495122,-26.4418155436,13.2586389408));
#97209=CARTESIAN_POINT('Ctrl Pts',(9.20832565648,-26.534489123,13.281014498));
#97210=CARTESIAN_POINT('Ctrl Pts',(9.03207275784,-26.2094852035,12.9888169711));
#97211=CARTESIAN_POINT('Ctrl Pts',(9.09749481749,-26.197804545,13.0669613638));
#97212=CARTESIAN_POINT('Ctrl Pts',(9.14338431009,-26.2207373383,13.1662307438));
#97213=CARTESIAN_POINT('Ctrl Pts',(9.15318354628,-26.2817510699,13.2674823288));
#97214=CARTESIAN_POINT('Ctrl Pts',(9.12391877788,-26.3632427792,13.341998513));
#97215=CARTESIAN_POINT('Ctrl Pts',(9.06936730061,-26.4447345097,13.3808551065));
#97216=CARTESIAN_POINT('Ctrl Pts',(8.97065416936,-26.1347652578,13.0157974347));
#97217=CARTESIAN_POINT('Ctrl Pts',(9.04345996357,-26.1233054476,13.0914671212));
#97218=CARTESIAN_POINT('Ctrl Pts',(9.08892654614,-26.1370041575,13.1967048874));
#97219=CARTESIAN_POINT('Ctrl Pts',(9.08730678255,-26.1793863705,13.3119583562));
#97220=CARTESIAN_POINT('Ctrl Pts',(9.03899779297,-26.2373408339,13.4022057303));
#97221=CARTESIAN_POINT('Ctrl Pts',(8.96418223747,-26.2952952698,13.4544010418));
#97222=CARTESIAN_POINT('Ctrl Pts',(8.9450884596,-26.0844303721,13.0266425468));
#97223=CARTESIAN_POINT('Ctrl Pts',(9.02199368194,-26.0754916974,13.1005323275));
#97224=CARTESIAN_POINT('Ctrl Pts',(9.0679762798,-26.0842677714,13.2078657435));
#97225=CARTESIAN_POINT('Ctrl Pts',(9.06149508662,-26.113583452,13.3291454014));
#97226=CARTESIAN_POINT('Ctrl Pts',(9.00457191343,-26.1541045198,13.4263466133));
#97227=CARTESIAN_POINT('Ctrl Pts',(8.92059308555,-26.1946255531,13.4844114062));
#97228=CARTESIAN_POINT('Ctrl Pts',(8.93233349646,-26.0293225561,13.0320605967));
#97229=CARTESIAN_POINT('Ctrl Pts',(9.0112864001,-26.0248786653,13.1050619605));
#97230=CARTESIAN_POINT('Ctrl Pts',(9.05753156729,-26.0292813737,13.2134376054));
#97231=CARTESIAN_POINT('Ctrl Pts',(9.04862484094,-26.0439316,13.3377236529));
#97232=CARTESIAN_POINT('Ctrl Pts',(8.98739853023,-26.0641705484,13.4383975561));
#97233=CARTESIAN_POINT('Ctrl Pts',(8.89884287263,-26.0844094969,13.4993947332));
#97234=CARTESIAN_POINT('Ctrl Pts',(8.93233349645,-25.9742356128,13.0320605967));
#97235=CARTESIAN_POINT('Ctrl Pts',(9.0112864001,-25.9742356128,13.1050619605));
#97236=CARTESIAN_POINT('Ctrl Pts',(9.05753156728,-25.9742356128,13.2134376055));
#97237=CARTESIAN_POINT('Ctrl Pts',(9.04862484094,-25.9742356128,13.3377236529));
#97238=CARTESIAN_POINT('Ctrl Pts',(8.98739853023,-25.9742356128,13.4383975561));
#97239=CARTESIAN_POINT('Ctrl Pts',(8.89884287263,-25.9742356128,13.4993947332));
#97240=CARTESIAN_POINT('',(8.89884287263,-25.9742356128,13.4993947332));
#97241=CARTESIAN_POINT('Ctrl Pts',(8.89884287263,-25.9742356128,13.4993947332));
#97242=CARTESIAN_POINT('Ctrl Pts',(8.91298306467026,-25.9742356128,13.4896549625125));
#97243=CARTESIAN_POINT('Ctrl Pts',(8.92628553401168,-25.9742356128,13.4786970415768));
#97244=CARTESIAN_POINT('Ctrl Pts',(8.93854791254593,-25.9742356128,13.4666811475669));
#97245=CARTESIAN_POINT('Ctrl Pts',(8.95104535408271,-25.9742356128,13.4544349155262));
#97246=CARTESIAN_POINT('Ctrl Pts',(8.96246226321512,-25.9742356128,13.4410901641476));
#97247=CARTESIAN_POINT('Ctrl Pts',(8.97262533430588,-25.9742356128,13.4268518558005));
#97248=CARTESIAN_POINT('Ctrl Pts',(8.98311909131686,-25.9742356128,13.4121502614983));
#97249=CARTESIAN_POINT('Ctrl Pts',(8.99227578537047,-25.9742356128,13.3964964516728));
#97250=CARTESIAN_POINT('Ctrl Pts',(8.99995175024907,-25.9742356128,13.3801470495469));
#97251=CARTESIAN_POINT('Ctrl Pts',(9.00766424539377,-25.9742356128,13.3637198398725));
#97252=CARTESIAN_POINT('Ctrl Pts',(9.01388179530927,-25.9742356128,13.3465910269051));
#97253=CARTESIAN_POINT('Ctrl Pts',(9.0185081506613,-25.9742356128,13.3290433912322));
#97254=CARTESIAN_POINT('Ctrl Pts',(9.02324515897379,-25.9742356128,13.3110760519938));
#97255=CARTESIAN_POINT('Ctrl Pts',(9.02631368963526,-25.9742356128,13.2926702667125));
#97256=CARTESIAN_POINT('Ctrl Pts',(9.02766503882281,-25.9742356128,13.274143441584));
#97257=CARTESIAN_POINT('Ctrl Pts',(9.0289486472493,-25.9742356128,13.2565453336559));
#97258=CARTESIAN_POINT('Ctrl Pts',(9.02868389097897,-25.9742356128,13.2388306328017));
#97259=CARTESIAN_POINT('Ctrl Pts',(9.02687144828272,-25.9742356128,13.2212742225973));
#97260=CARTESIAN_POINT('Ctrl Pts',(9.02502174785923,-25.9742356128,13.2033569116351));
#97261=CARTESIAN_POINT('Ctrl Pts',(9.02155985184751,-25.9742356128,13.1856052086565));
#97262=CARTESIAN_POINT('Ctrl Pts',(9.01653597905922,-25.9742356128,13.168306927222));
#97263=CARTESIAN_POINT('Ctrl Pts',(9.01158677833036,-25.9742356128,13.151265757851));
#97264=CARTESIAN_POINT('Ctrl Pts',(9.0051217696928,-25.9742356128,13.1346651906981));
#97265=CARTESIAN_POINT('Ctrl Pts',(8.9972370966015,-25.9742356128,13.1187670484391));
#97266=CARTESIAN_POINT('Ctrl Pts',(8.98917398112835,-25.9742356128,13.1025091065614));
#97267=CARTESIAN_POINT('Ctrl Pts',(8.97962599034423,-25.9742356128,13.086986455719));
#97268=CARTESIAN_POINT('Ctrl Pts',(8.96874817699059,-25.9742356128,13.0724552782259));
#97269=CARTESIAN_POINT('Ctrl Pts',(8.95848641872981,-25.9742356128,13.05874706079));
#97270=CARTESIAN_POINT('Ctrl Pts',(8.94704161419982,-25.9742356128,13.0459214436467));
#97271=CARTESIAN_POINT('Ctrl Pts',(8.9345873676507,-25.9742356128,13.0341661661072));
#97272=CARTESIAN_POINT('Ctrl Pts',(8.93383968856693,-25.9742356128,13.0334604489765));
#97273=CARTESIAN_POINT('Ctrl Pts',(8.93308838402742,-25.9742356128,13.0327585801828));
#97274=CARTESIAN_POINT('Ctrl Pts',(8.93233349645,-25.9742356128,13.0320605967));
#97275=CARTESIAN_POINT('Ctrl Pts',(9.40585253196699,-26.5742356128001,13.1350808874316));
#97276=CARTESIAN_POINT('Ctrl Pts',(9.38966886904336,-26.5742356625068,13.1472052249601));
#97277=CARTESIAN_POINT('Ctrl Pts',(9.37371043414577,-26.5732883695804,13.1591121368475));
#97278=CARTESIAN_POINT('Ctrl Pts',(9.35792283466795,-26.5714573040172,13.1708460778927));
#97279=CARTESIAN_POINT('Ctrl Pts',(9.34201605619545,-26.569612415925,13.1826685972742));
#97280=CARTESIAN_POINT('Ctrl Pts',(9.32628204370353,-26.5668701774511,13.1943160189337));
#97281=CARTESIAN_POINT('Ctrl Pts',(9.31066243960798,-26.5632416337301,13.2058344298026));
#97282=CARTESIAN_POINT('Ctrl Pts',(9.29515443644995,-26.5596390156906,13.2172705424618));
#97283=CARTESIAN_POINT('Ctrl Pts',(9.27975857422437,-26.5551624841021,13.2285799346777));
#97284=CARTESIAN_POINT('Ctrl Pts',(9.2644247047449,-26.5497730925338,13.2398012826113));
#97285=CARTESIAN_POINT('Ctrl Pts',(9.24921727962928,-26.5444281423369,13.2509300983759));
#97286=CARTESIAN_POINT('Ctrl Pts',(9.23407016532093,-26.5381851359198,13.2619727680672));
#97287=CARTESIAN_POINT('Ctrl Pts',(9.2189509255191,-26.5309600288552,13.2729539975724));
#97288=CARTESIAN_POINT('Ctrl Pts',(9.20382905634151,-26.5237336652776,13.2839371368152));
#97289=CARTESIAN_POINT('Ctrl Pts',(9.18918039767918,-26.5157377018366,13.2945354690637));
#97290=CARTESIAN_POINT('Ctrl Pts',(9.17494003359809,-26.5069897570663,13.3048032283136));
#97291=CARTESIAN_POINT('Ctrl Pts',(9.16059836413125,-26.4981795797635,13.3151440319958));
#97292=CARTESIAN_POINT('Ctrl Pts',(9.1466701415747,-26.4886063214309,13.3251499910549));
#97293=CARTESIAN_POINT('Ctrl Pts',(9.13310430195239,-26.4782388663181,13.3348638296197));
#97294=CARTESIAN_POINT('Ctrl Pts',(9.11953846233007,-26.4678714112053,13.3445776681844));
#97295=CARTESIAN_POINT('Ctrl Pts',(9.10633428546738,-26.4567093462435,13.3539998486706));
#97296=CARTESIAN_POINT('Ctrl Pts',(9.09346630996625,-26.4446784843961,13.3631536894615));
#97297=CARTESIAN_POINT('Ctrl Pts',(9.08047306334464,-26.4325305008194,13.3723966438733));
#97298=CARTESIAN_POINT('Ctrl Pts',(9.06782160736129,-26.4194959284248,13.3813666470324));
#97299=CARTESIAN_POINT('Ctrl Pts',(9.0555219142915,-26.4054564922348,13.3900613629745));
#97300=CARTESIAN_POINT('Ctrl Pts',(9.04333267047346,-26.3915431279079,13.3986780017756));
#97301=CARTESIAN_POINT('Ctrl Pts',(9.03188529279735,-26.3770877111105,13.4067442529712));
#97302=CARTESIAN_POINT('Ctrl Pts',(9.0211058886148,-26.3620851591429,13.4143208599837));
#97303=CARTESIAN_POINT('Ctrl Pts',(9.01063047203914,-26.3475056908441,13.4216838007681));
#97304=CARTESIAN_POINT('Ctrl Pts',(9.00078546904118,-26.3324087757691,13.4285845585318));
#97305=CARTESIAN_POINT('Ctrl Pts',(8.9915296376939,-26.316749732984,13.4350584629122));
#97306=CARTESIAN_POINT('Ctrl Pts',(8.98237304571567,-26.3012585836562,13.4414629552472));
#97307=CARTESIAN_POINT('Ctrl Pts',(8.97379258055418,-26.2852166573475,13.4474499888569));
#97308=CARTESIAN_POINT('Ctrl Pts',(8.96578137748102,-26.2685508639815,13.4530295650986));
#97309=CARTESIAN_POINT('Ctrl Pts',(8.95797597478179,-26.2523131993841,13.4584658072035));
#97310=CARTESIAN_POINT('Ctrl Pts',(8.95071060864188,-26.2354825818213,13.4635154704097));
#97311=CARTESIAN_POINT('Ctrl Pts',(8.9440164384977,-26.2179729998285,13.4681611210768));
#97312=CARTESIAN_POINT('Ctrl Pts',(8.94308638265781,-26.2155403026254,13.468806565462));
#97313=CARTESIAN_POINT('Ctrl Pts',(8.94216741815707,-26.2130944800201,13.4694441650684));
#97314=CARTESIAN_POINT('Ctrl Pts',(8.94125969379736,-26.2106352851941,13.4700738273255));
#97315=CARTESIAN_POINT('Ctrl Pts',(8.93349674327698,-26.1896040023491,13.4754587626243));
#97316=CARTESIAN_POINT('Ctrl Pts',(8.92683498762293,-26.1683122326554,13.4800697405241));
#97317=CARTESIAN_POINT('Ctrl Pts',(8.92122702740422,-26.1467792344255,13.4839469960848));
#97318=CARTESIAN_POINT('Ctrl Pts',(8.9155694983306,-26.1250559056613,13.4878585227728));
#97319=CARTESIAN_POINT('Ctrl Pts',(8.9109841011639,-26.1030857806081,13.4910235212305));
#97320=CARTESIAN_POINT('Ctrl Pts',(8.90746043306424,-26.0808653513723,13.4934542237138));
#97321=CARTESIAN_POINT('Ctrl Pts',(8.9039681996182,-26.0588431506521,13.4958632418931));
#97322=CARTESIAN_POINT('Ctrl Pts',(8.90151881605978,-26.0365736279148,13.4975510147087));
#97323=CARTESIAN_POINT('Ctrl Pts',(8.90014240237732,-26.014051170286,13.4984994019142));
#97324=CARTESIAN_POINT('Ctrl Pts',(8.89933657923613,-26.0008653688186,13.4990546364101));
#97325=CARTESIAN_POINT('Ctrl Pts',(8.89889929429057,-25.9875929284109,13.4993558699346));
#97326=CARTESIAN_POINT('Ctrl Pts',(8.89884287263,-25.9742356128,13.4993947332));
#97327=CARTESIAN_POINT('Origin',(8.72866611926,-27.9742356128,13.252332246));
#97328=CARTESIAN_POINT('',(8.89884287263,-27.8242356128,13.4993947332));
#97329=CARTESIAN_POINT('Origin',(-4.21848174452E-16,-27.8242356128,0.580061096523));
#98288=UNCERTAINTY_MEASURE_WITH_UNIT(LENGTH_MEASURE(0.01),#98303,
'DISTANCE_ACCURACY_VALUE',
'Maximum model space distance between geometric entities at asserted c
onnectivities');
#98290=UNCERTAINTY_MEASURE_WITH_UNIT(LENGTH_MEASURE(0.01),#98303,
'DISTANCE_ACCURACY_VALUE',
'Maximum model space distance between geometric entities at asserted c
onnectivities');
#98300=(
GEOMETRIC_REPRESENTATION_CONTEXT(3)
GLOBAL_UNCERTAINTY_ASSIGNED_CONTEXT((#98288))
GLOBAL_UNIT_ASSIGNED_CONTEXT((#98303,#98305,#98306))
REPRESENTATION_CONTEXT('','3D')
);
#98302=(
GEOMETRIC_REPRESENTATION_CONTEXT(3)
GLOBAL_UNCERTAINTY_ASSIGNED_CONTEXT((#98290))
GLOBAL_UNIT_ASSIGNED_CONTEXT((#98303,#98305,#98306))
REPRESENTATION_CONTEXT('','3D')
);
#98303=(
LENGTH_UNIT()
NAMED_UNIT(*)
SI_UNIT(.MILLI.,.METRE.)
);
#98305=(
NAMED_UNIT(*)
PLANE_ANGLE_UNIT()
SI_UNIT($,.RADIAN.)
);
#98306=(
NAMED_UNIT(*)
SI_UNIT($,.STERADIAN.)
SOLID_ANGLE_UNIT()
);
#98316=SHAPE_DEFINITION_REPRESENTATION(#98327,#98348);
#98327=PRODUCT_DEFINITION_SHAPE('',$,#98360);
#98348=SHAPE_REPRESENTATION('',(#38088),#98300);
#98350=PRODUCT_DEFINITION_CONTEXT('part definition',#98385,'design');
#98360=PRODUCT_DEFINITION('Movable Ceramic Disc','Movable Ceramic Disc',
#98371,#98350);
#98371=PRODUCT_DEFINITION_FORMATION('',$,#98396);
#98385=APPLICATION_CONTEXT(
'Core Data for Automotive Mechanical Design Process');
#98386=PRODUCT_CONTEXT('part definition',#98385,'mechanical');
#98396=PRODUCT('Movable Ceramic Disc','Movable Ceramic Disc',$,(#98386));
#98399=PRESENTATION_STYLE_ASSIGNMENT((#98401));
#98401=SURFACE_STYLE_USAGE(.BOTH.,#98403);
#98403=SURFACE_SIDE_STYLE('',(#98405));
#98405=SURFACE_STYLE_FILL_AREA(#98407);
#98407=FILL_AREA_STYLE('Opaque(202,209,238)',(#98409));
#98409=FILL_AREA_STYLE_COLOUR('Opaque(202,209,238)',#98411);
#98411=COLOUR_RGB('Opaque(202,209,238)', 0.31764706, 0.68627451, 0.89019608);
ENDSEC;
END-ISO-10303-21;
